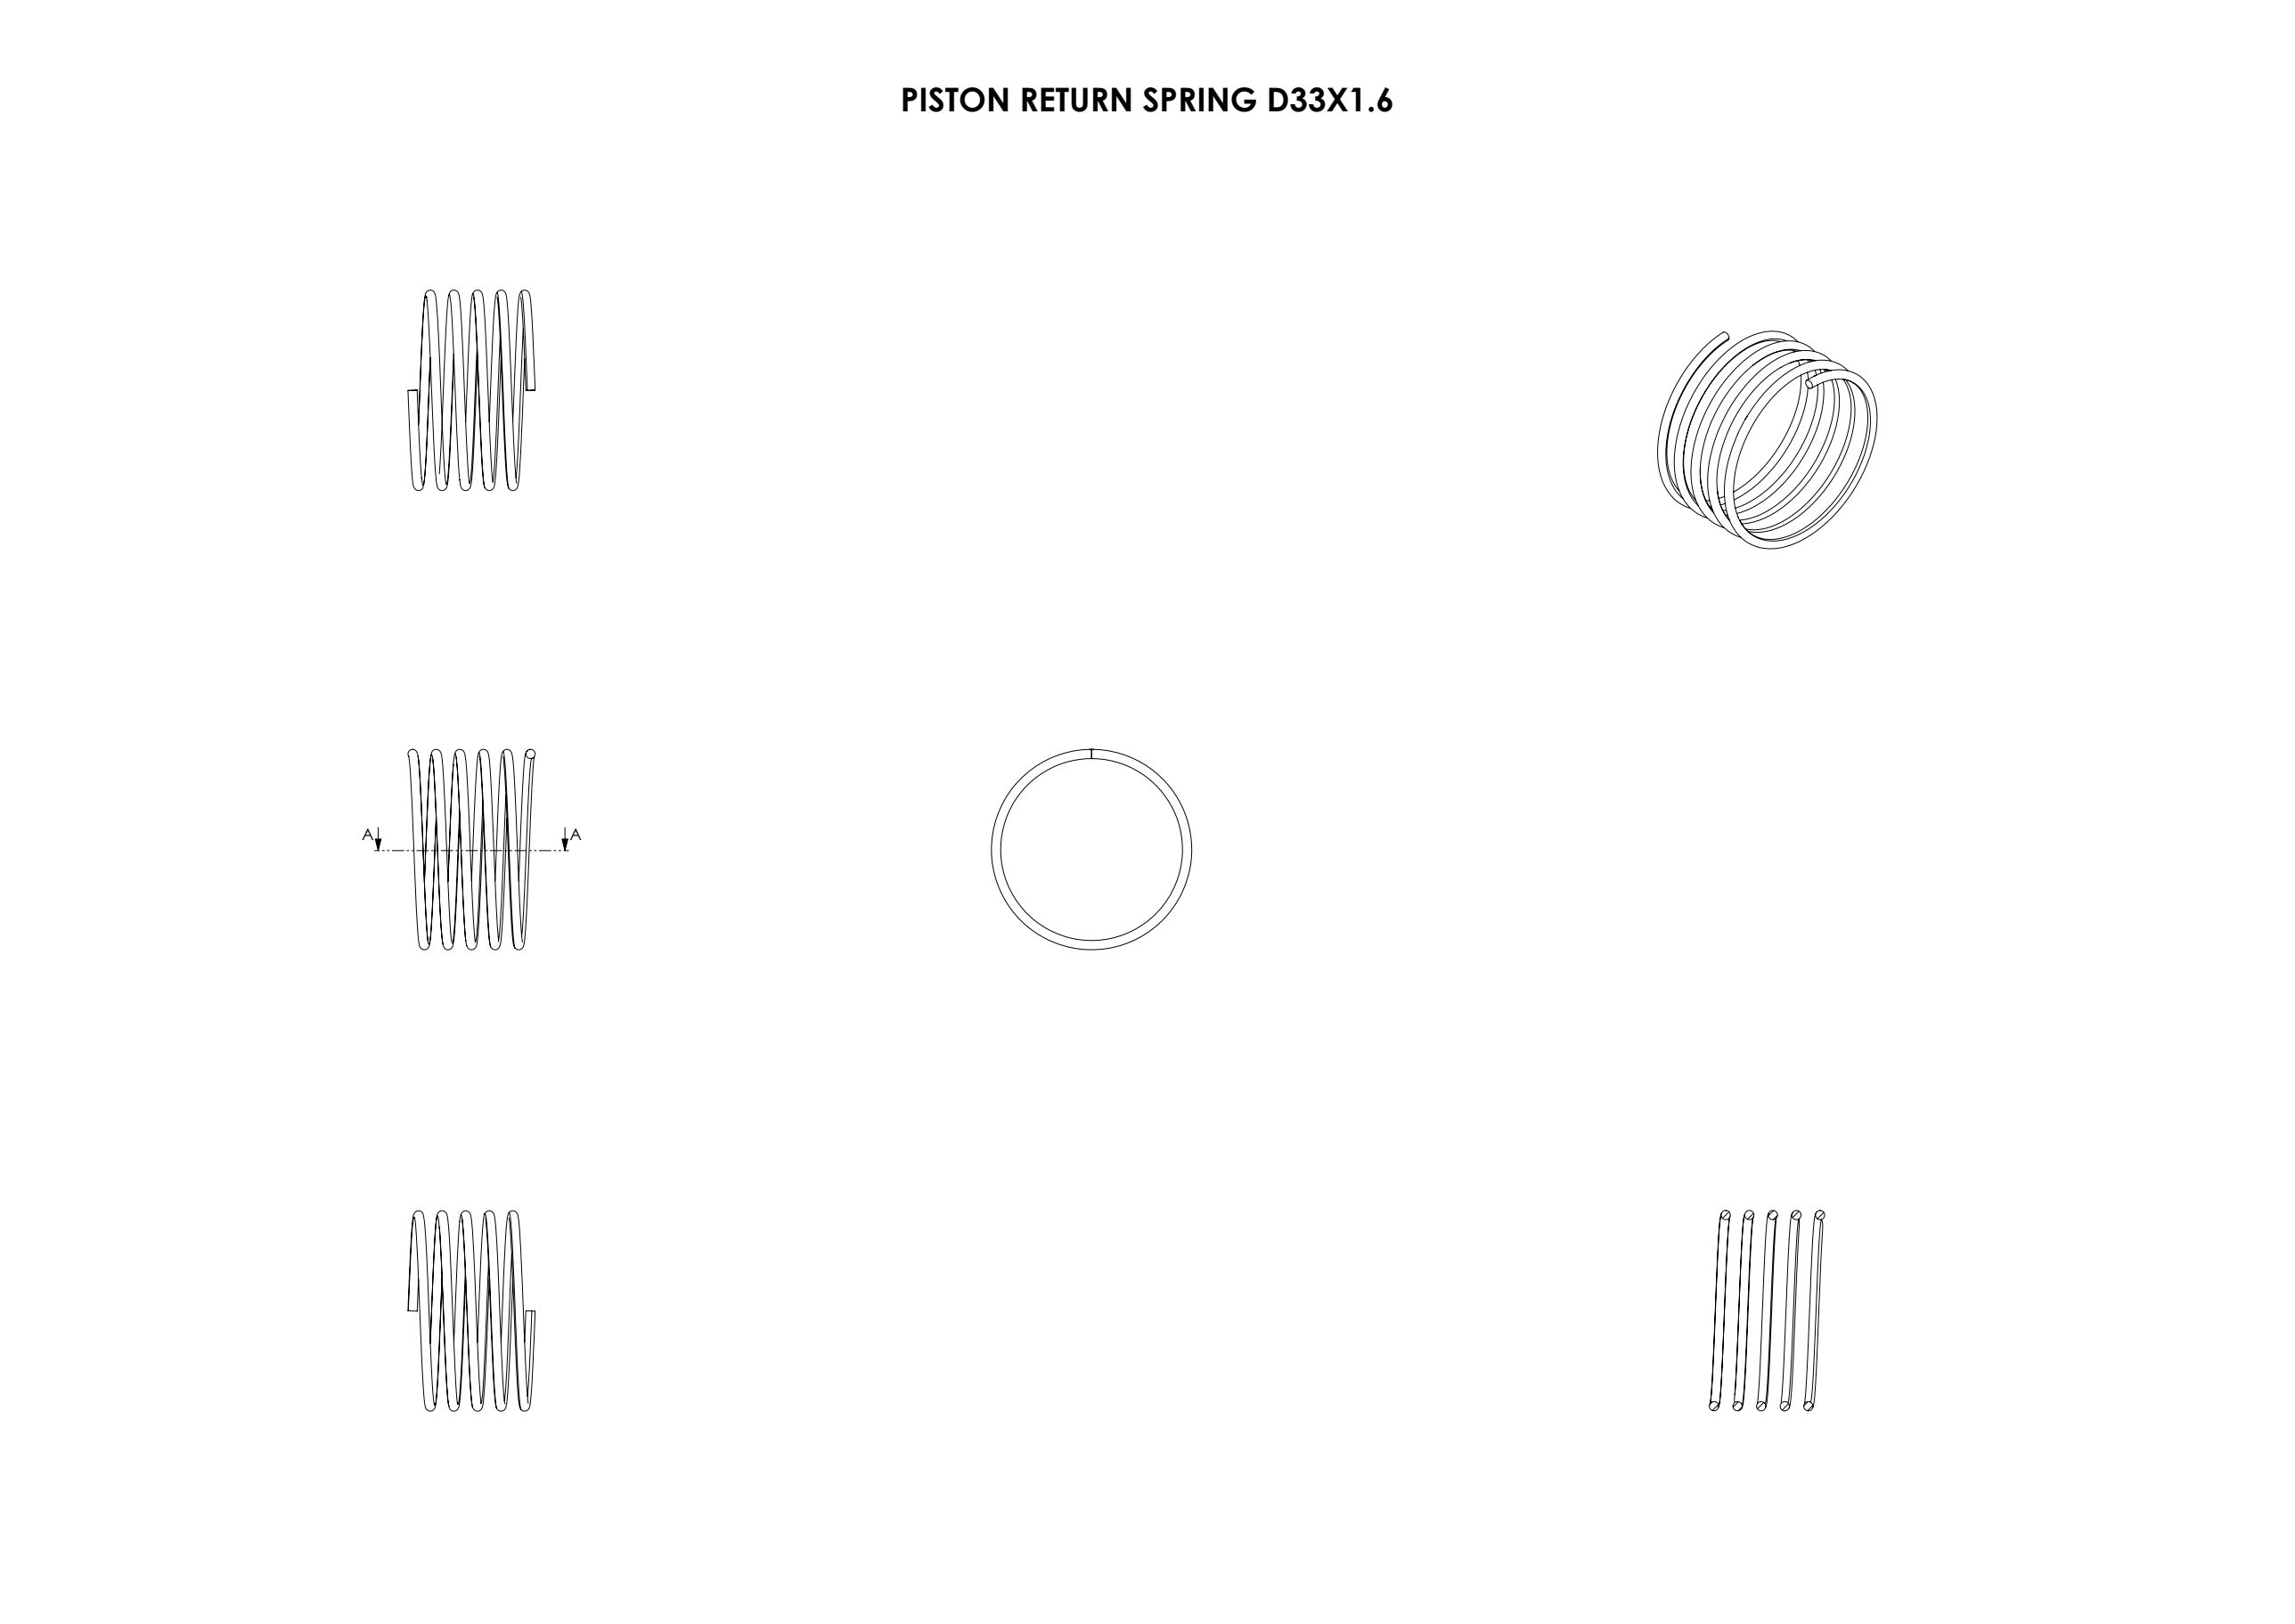
ISO-10303-21;
HEADER;
/* Generated by software containing ST-Developer
 * from STEP Tools, Inc. (www.steptools.com) 
 */

FILE_DESCRIPTION(
/* description */ (''),
/* implementation_level */ '2;1');

FILE_NAME(
/* name */ '04_Piston_Return_Spring_D33x1.6.step',
/* time_stamp */ '2026-10-26T03:55:20-07:00',
/* author */ (''),
/* organization */ (''),
/* preprocessor_version */ 'ST-DEVELOPER v20.2',
/* originating_system */ 'Autodesk Translation Framework v15.15.0.0',
/* authorisation */ '');

FILE_SCHEMA (('AUTOMOTIVE_DESIGN { 1 0 10303 214 3 1 1 }'));
ENDSEC;

DATA;
#10=MECHANICAL_DESIGN_GEOMETRIC_PRESENTATION_REPRESENTATION('',(#178),#45236);
#138=SHAPE_REPRESENTATION_RELATIONSHIP('SRR','None',#45317,#158);
#158=ADVANCED_BREP_SHAPE_REPRESENTATION('',(#198),#45219);
#178=STYLED_ITEM('',(#45484),#198);
#198=MANIFOLD_SOLID_BREP('Body1',#16520);
#484=B_SPLINE_CURVE_WITH_KNOTS('',3,(#32149,#32150,#32151,#32152,#32153,
#32154,#32155,#32156,#32157,#32158,#32159,#32160,#32161,#32162,#32163,#32164,
#32165,#32166,#32167,#32168,#32169,#32170,#32171,#32172,#32173,#32174,#32175,
#32176,#32177,#32178,#32179,#32180,#32181,#32182,#32183,#32184,#32185,#32186,
#32187,#32188,#32189,#32190,#32191,#32192,#32193,#32194,#32195,#32196,#32197,
#32198,#32199,#32200,#32201,#32202,#32203,#32204,#32205,#32206,#32207,#32208,
#32209,#32210,#32211,#32212,#32213,#32214,#32215,#32216,#32217,#32218,#32219,
#32220,#32221,#32222,#32223),.UNSPECIFIED.,.F.,.F.,(4,1,1,1,1,1,1,1,1,1,
1,1,1,1,1,1,1,1,1,1,1,1,1,1,1,1,1,1,1,1,1,1,1,1,1,1,1,1,1,1,1,1,1,1,1,1,
1,1,1,1,1,1,1,1,1,1,1,1,1,1,1,1,1,1,1,1,1,1,1,1,1,1,4),(0.,0.00892857142857143,
0.0178571428571429,0.0357142857142857,0.0535714285714286,0.0714285714285714,
0.0892857142857143,0.107142857142857,0.116071428571429,0.125,0.133928571428571,
0.142857142857143,0.154761904761905,0.166666666666667,0.178571428571429,
0.19047619047619,0.202380952380952,0.214285714285714,0.232142857142857,
0.25,0.267857142857143,0.285714285714286,0.303571428571429,0.321428571428571,
0.339285714285714,0.357142857142857,0.376984126984127,0.380952380952381,
0.392857142857143,0.404761904761905,0.416666666666667,0.428571428571429,
0.44047619047619,0.452380952380952,0.464285714285714,0.476190476190476,
0.492063492063492,0.5,0.517857142857143,0.535714285714286,0.553571428571429,
0.571428571428571,0.589285714285714,0.607142857142857,0.625,0.642857142857143,
0.654761904761905,0.666666666666667,0.678571428571428,0.69047619047619,
0.702380952380952,0.714285714285714,0.726190476190476,0.738095238095238,
0.75,0.761904761904762,0.773809523809524,0.785714285714286,0.797619047619047,
0.809523809523809,0.821428571428571,0.833333333333333,0.845238095238095,
0.857142857142857,0.875,0.892857142857143,0.910714285714286,0.928571428571429,
0.946428571428571,0.964285714285714,0.982142857142857,0.991071428571429,
1.),.UNSPECIFIED.);
#857=B_SPLINE_SURFACE_WITH_KNOTS('',3,3,((#31396,#31397,#31398,#31399,#31400,
#31401,#31402,#31403,#31404,#31405,#31406,#31407,#31408,#31409,#31410,#31411,
#31412,#31413,#31414,#31415,#31416,#31417,#31418,#31419,#31420,#31421,#31422,
#31423,#31424,#31425,#31426,#31427,#31428,#31429,#31430,#31431,#31432,#31433,
#31434,#31435,#31436,#31437,#31438,#31439,#31440,#31441,#31442,#31443,#31444,
#31445,#31446,#31447,#31448,#31449,#31450,#31451,#31452,#31453,#31454,#31455,
#31456,#31457,#31458,#31459,#31460,#31461,#31462,#31463,#31464,#31465,#31466,
#31467,#31468,#31469,#31470),(#31471,#31472,#31473,#31474,#31475,#31476,
#31477,#31478,#31479,#31480,#31481,#31482,#31483,#31484,#31485,#31486,#31487,
#31488,#31489,#31490,#31491,#31492,#31493,#31494,#31495,#31496,#31497,#31498,
#31499,#31500,#31501,#31502,#31503,#31504,#31505,#31506,#31507,#31508,#31509,
#31510,#31511,#31512,#31513,#31514,#31515,#31516,#31517,#31518,#31519,#31520,
#31521,#31522,#31523,#31524,#31525,#31526,#31527,#31528,#31529,#31530,#31531,
#31532,#31533,#31534,#31535,#31536,#31537,#31538,#31539,#31540,#31541,#31542,
#31543,#31544,#31545),(#31546,#31547,#31548,#31549,#31550,#31551,#31552,
#31553,#31554,#31555,#31556,#31557,#31558,#31559,#31560,#31561,#31562,#31563,
#31564,#31565,#31566,#31567,#31568,#31569,#31570,#31571,#31572,#31573,#31574,
#31575,#31576,#31577,#31578,#31579,#31580,#31581,#31582,#31583,#31584,#31585,
#31586,#31587,#31588,#31589,#31590,#31591,#31592,#31593,#31594,#31595,#31596,
#31597,#31598,#31599,#31600,#31601,#31602,#31603,#31604,#31605,#31606,#31607,
#31608,#31609,#31610,#31611,#31612,#31613,#31614,#31615,#31616,#31617,#31618,
#31619,#31620),(#31621,#31622,#31623,#31624,#31625,#31626,#31627,#31628,
#31629,#31630,#31631,#31632,#31633,#31634,#31635,#31636,#31637,#31638,#31639,
#31640,#31641,#31642,#31643,#31644,#31645,#31646,#31647,#31648,#31649,#31650,
#31651,#31652,#31653,#31654,#31655,#31656,#31657,#31658,#31659,#31660,#31661,
#31662,#31663,#31664,#31665,#31666,#31667,#31668,#31669,#31670,#31671,#31672,
#31673,#31674,#31675,#31676,#31677,#31678,#31679,#31680,#31681,#31682,#31683,
#31684,#31685,#31686,#31687,#31688,#31689,#31690,#31691,#31692,#31693,#31694,
#31695),(#31696,#31697,#31698,#31699,#31700,#31701,#31702,#31703,#31704,
#31705,#31706,#31707,#31708,#31709,#31710,#31711,#31712,#31713,#31714,#31715,
#31716,#31717,#31718,#31719,#31720,#31721,#31722,#31723,#31724,#31725,#31726,
#31727,#31728,#31729,#31730,#31731,#31732,#31733,#31734,#31735,#31736,#31737,
#31738,#31739,#31740,#31741,#31742,#31743,#31744,#31745,#31746,#31747,#31748,
#31749,#31750,#31751,#31752,#31753,#31754,#31755,#31756,#31757,#31758,#31759,
#31760,#31761,#31762,#31763,#31764,#31765,#31766,#31767,#31768,#31769,#31770),
(#31771,#31772,#31773,#31774,#31775,#31776,#31777,#31778,#31779,#31780,
#31781,#31782,#31783,#31784,#31785,#31786,#31787,#31788,#31789,#31790,#31791,
#31792,#31793,#31794,#31795,#31796,#31797,#31798,#31799,#31800,#31801,#31802,
#31803,#31804,#31805,#31806,#31807,#31808,#31809,#31810,#31811,#31812,#31813,
#31814,#31815,#31816,#31817,#31818,#31819,#31820,#31821,#31822,#31823,#31824,
#31825,#31826,#31827,#31828,#31829,#31830,#31831,#31832,#31833,#31834,#31835,
#31836,#31837,#31838,#31839,#31840,#31841,#31842,#31843,#31844,#31845),
(#31846,#31847,#31848,#31849,#31850,#31851,#31852,#31853,#31854,#31855,
#31856,#31857,#31858,#31859,#31860,#31861,#31862,#31863,#31864,#31865,#31866,
#31867,#31868,#31869,#31870,#31871,#31872,#31873,#31874,#31875,#31876,#31877,
#31878,#31879,#31880,#31881,#31882,#31883,#31884,#31885,#31886,#31887,#31888,
#31889,#31890,#31891,#31892,#31893,#31894,#31895,#31896,#31897,#31898,#31899,
#31900,#31901,#31902,#31903,#31904,#31905,#31906,#31907,#31908,#31909,#31910,
#31911,#31912,#31913,#31914,#31915,#31916,#31917,#31918,#31919,#31920),
(#31921,#31922,#31923,#31924,#31925,#31926,#31927,#31928,#31929,#31930,
#31931,#31932,#31933,#31934,#31935,#31936,#31937,#31938,#31939,#31940,#31941,
#31942,#31943,#31944,#31945,#31946,#31947,#31948,#31949,#31950,#31951,#31952,
#31953,#31954,#31955,#31956,#31957,#31958,#31959,#31960,#31961,#31962,#31963,
#31964,#31965,#31966,#31967,#31968,#31969,#31970,#31971,#31972,#31973,#31974,
#31975,#31976,#31977,#31978,#31979,#31980,#31981,#31982,#31983,#31984,#31985,
#31986,#31987,#31988,#31989,#31990,#31991,#31992,#31993,#31994,#31995),
(#31996,#31997,#31998,#31999,#32000,#32001,#32002,#32003,#32004,#32005,
#32006,#32007,#32008,#32009,#32010,#32011,#32012,#32013,#32014,#32015,#32016,
#32017,#32018,#32019,#32020,#32021,#32022,#32023,#32024,#32025,#32026,#32027,
#32028,#32029,#32030,#32031,#32032,#32033,#32034,#32035,#32036,#32037,#32038,
#32039,#32040,#32041,#32042,#32043,#32044,#32045,#32046,#32047,#32048,#32049,
#32050,#32051,#32052,#32053,#32054,#32055,#32056,#32057,#32058,#32059,#32060,
#32061,#32062,#32063,#32064,#32065,#32066,#32067,#32068,#32069,#32070),
(#32071,#32072,#32073,#32074,#32075,#32076,#32077,#32078,#32079,#32080,
#32081,#32082,#32083,#32084,#32085,#32086,#32087,#32088,#32089,#32090,#32091,
#32092,#32093,#32094,#32095,#32096,#32097,#32098,#32099,#32100,#32101,#32102,
#32103,#32104,#32105,#32106,#32107,#32108,#32109,#32110,#32111,#32112,#32113,
#32114,#32115,#32116,#32117,#32118,#32119,#32120,#32121,#32122,#32123,#32124,
#32125,#32126,#32127,#32128,#32129,#32130,#32131,#32132,#32133,#32134,#32135,
#32136,#32137,#32138,#32139,#32140,#32141,#32142,#32143,#32144,#32145)),
 .UNSPECIFIED.,.T.,.F.,.F.,(4,1,1,1,1,1,1,4),(4,1,1,1,1,1,1,1,1,1,1,1,1,
1,1,1,1,1,1,1,1,1,1,1,1,1,1,1,1,1,1,1,1,1,1,1,1,1,1,1,1,1,1,1,1,1,1,1,1,
1,1,1,1,1,1,1,1,1,1,1,1,1,1,1,1,1,1,1,1,1,1,1,4),(-3.14159265358979,-2.24399475256414,
-1.34639685153848,-0.448798950512828,0.448798950512828,1.34639685153848,
2.24399475256414,3.14159265358979),(0.,0.00892857142857143,0.0178571428571429,
0.0357142857142857,0.0535714285714286,0.0714285714285714,0.0892857142857143,
0.107142857142857,0.116071428571429,0.125,0.133928571428571,0.142857142857143,
0.154761904761905,0.166666666666667,0.178571428571429,0.19047619047619,
0.202380952380952,0.214285714285714,0.232142857142857,0.25,0.267857142857143,
0.285714285714286,0.303571428571429,0.321428571428571,0.339285714285714,
0.357142857142857,0.376984126984127,0.380952380952381,0.392857142857143,
0.404761904761905,0.416666666666667,0.428571428571429,0.44047619047619,
0.452380952380952,0.464285714285714,0.476190476190476,0.492063492063492,
0.5,0.517857142857143,0.535714285714286,0.553571428571429,0.571428571428571,
0.589285714285714,0.607142857142857,0.625,0.642857142857143,0.654761904761905,
0.666666666666667,0.678571428571428,0.69047619047619,0.702380952380952,
0.714285714285714,0.726190476190476,0.738095238095238,0.75,0.761904761904762,
0.773809523809524,0.785714285714286,0.797619047619047,0.809523809523809,
0.821428571428571,0.833333333333333,0.845238095238095,0.857142857142857,
0.875,0.892857142857143,0.910714285714286,0.928571428571429,0.946428571428571,
0.964285714285714,0.982142857142857,0.991071428571429,1.),.UNSPECIFIED.);
#1130=PLANE('',#17150);
#1131=PLANE('',#17151);
#2088=FACE_OUTER_BOUND('',#3086,.T.);
#2089=FACE_OUTER_BOUND('',#3087,.T.);
#2090=FACE_OUTER_BOUND('',#3088,.T.);
#3086=EDGE_LOOP('',(#12128,#12129,#12130,#12131));
#3087=EDGE_LOOP('',(#12132));
#3088=EDGE_LOOP('',(#12133));
#6661=CIRCLE('',#17148,0.8);
#6662=CIRCLE('',#17149,0.8);
#7377=VERTEX_POINT('',#32146);
#7378=VERTEX_POINT('',#32148);
#9127=EDGE_CURVE('',#7377,#7377,#6661,.T.);
#9128=EDGE_CURVE('',#7377,#7378,#484,.T.);
#9129=EDGE_CURVE('',#7378,#7378,#6662,.T.);
#12128=ORIENTED_EDGE('',*,*,#9127,.T.);
#12129=ORIENTED_EDGE('',*,*,#9128,.T.);
#12130=ORIENTED_EDGE('',*,*,#9129,.F.);
#12131=ORIENTED_EDGE('',*,*,#9128,.F.);
#12132=ORIENTED_EDGE('',*,*,#9129,.T.);
#12133=ORIENTED_EDGE('',*,*,#9127,.F.);
#15816=ADVANCED_FACE('',(#2088),#857,.T.);
#15817=ADVANCED_FACE('',(#2089),#1130,.T.);
#15818=ADVANCED_FACE('',(#2090),#1131,.F.);
#16520=CLOSED_SHELL('',(#15816,#15817,#15818));
#17147=AXIS2_PLACEMENT_3D('',#31395,#19181,#19182);
#17148=AXIS2_PLACEMENT_3D('',#32147,#19183,#19184);
#17149=AXIS2_PLACEMENT_3D('',#32224,#19185,#19186);
#17150=AXIS2_PLACEMENT_3D('',#32225,#19187,#19188);
#17151=AXIS2_PLACEMENT_3D('',#32226,#19189,#19190);
#19181=DIRECTION('axis',(0.,0.,1.));
#19182=DIRECTION('refdir',(1.,0.,0.));
#19183=DIRECTION('center_axis',(0.0385833407296796,-0.00185275719821836,
0.99925366804876));
#19184=DIRECTION('ref_axis',(-0.998103575378143,0.0479285502208167,0.0386277994596909));
#19185=DIRECTION('center_axis',(0.0385833409756958,0.0018527571775933,0.999253668039299));
#19186=DIRECTION('ref_axis',(-0.285673463027164,0.95828233937443,0.00925367846524069));
#19187=DIRECTION('center_axis',(0.0385833409756958,0.0018527571775933,0.999253668039299));
#19188=DIRECTION('ref_axis',(-0.285673463027164,0.95828233937443,0.00925367846524068));
#19189=DIRECTION('center_axis',(0.0385833407296796,-0.00185275719821836,
0.99925366804876));
#19190=DIRECTION('ref_axis',(-0.998103575378143,0.0479285502208167,0.0386277994596909));
#31395=CARTESIAN_POINT('',(0.,0.,0.));
#31396=CARTESIAN_POINT('Ctrl Pts',(69.6184828603025,16.4616571598233,-0.030902239567753));
#31397=CARTESIAN_POINT('Ctrl Pts',(69.6789219655699,16.458754897209,1.53438465601481));
#31398=CARTESIAN_POINT('Ctrl Pts',(69.7997830801149,16.0266321943109,4.57501994136558));
#31399=CARTESIAN_POINT('Ctrl Pts',(70.0414349064678,13.4941722421641,10.2617903021912));
#31400=CARTESIAN_POINT('Ctrl Pts',(70.3432064666604,7.54051932200945,15.5847054098009));
#31401=CARTESIAN_POINT('Ctrl Pts',(70.7049768750637,-1.90873983484295,17.1894487135762));
#31402=CARTESIAN_POINT('Ctrl Pts',(71.0663492060979,-10.7475553396686,13.525924310196));
#31403=CARTESIAN_POINT('Ctrl Pts',(71.4273437518671,-16.2818464768058,5.72657424978343));
#31404=CARTESIAN_POINT('Ctrl Pts',(71.7278512234343,-16.7210289894503,-2.21659997283488));
#31405=CARTESIAN_POINT('Ctrl Pts',(71.9680675578449,-14.5106197428725,-7.98557322489482));
#31406=CARTESIAN_POINT('Ctrl Pts',(72.1481344157904,-11.7288725172833,-11.6852538002611));
#31407=CARTESIAN_POINT('Ctrl Pts',(72.328106524648,-8.03024824250695,-14.4669696417765));
#31408=CARTESIAN_POINT('Ctrl Pts',(72.5279702250768,-3.22977654241172,-16.300670274406));
#31409=CARTESIAN_POINT('Ctrl Pts',(72.7476856540044,2.4587525001183,-16.5141747132305));
#31410=CARTESIAN_POINT('Ctrl Pts',(72.9872078330289,8.31673840998305,-14.4634243432854));
#31411=CARTESIAN_POINT('Ctrl Pts',(73.2265632969346,13.0163496494046,-10.4182667032949));
#31412=CARTESIAN_POINT('Ctrl Pts',(73.4657526686465,15.9141590581627,-4.93897396144999));
#31413=CARTESIAN_POINT('Ctrl Pts',(73.7047766516472,16.6034312776959,1.21397241511146));
#31414=CARTESIAN_POINT('Ctrl Pts',(73.9834458021771,14.7409225736484,8.19195097348461));
#31415=CARTESIAN_POINT('Ctrl Pts',(74.301651818573,9.13086318160831,14.4766680019069));
#31416=CARTESIAN_POINT('Ctrl Pts',(74.6592672763964,0.0266353994119735,
17.0966775050227));
#31417=CARTESIAN_POINT('Ctrl Pts',(75.016519558125,-9.06348425632334,14.4765973593132));
#31418=CARTESIAN_POINT('Ctrl Pts',(75.3734117874807,-15.3610417662207,7.42742367726323));
#31419=CARTESIAN_POINT('Ctrl Pts',(75.7299471567895,-16.9418739975217,-1.88122771580553));
#31420=CARTESIAN_POINT('Ctrl Pts',(76.0861289312927,-13.3290621410899,-10.5975142741848));
#31421=CARTESIAN_POINT('Ctrl Pts',(76.4419606933661,-5.64617345782912,-16.0463992053949));
#31422=CARTESIAN_POINT('Ctrl Pts',(76.810612386967,4.11087115606672,-16.6005218369866));
#31423=CARTESIAN_POINT('Ctrl Pts',(77.0868204963524,10.4484384772329,-12.8295775485076));
#31424=CARTESIAN_POINT('Ctrl Pts',(77.3234199677928,14.1464940116618,-8.0565595801055));
#31425=CARTESIAN_POINT('Ctrl Pts',(77.5073642434964,16.0558684975652,-3.69288655028273));
#31426=CARTESIAN_POINT('Ctrl Pts',(77.743715642047,16.2835727900373,2.42892269363191));
#31427=CARTESIAN_POINT('Ctrl Pts',(77.9799198273595,14.2624210045081,8.20410639070391));
#31428=CARTESIAN_POINT('Ctrl Pts',(78.2159782861261,10.2721221270508,12.8404255794219));
#31429=CARTESIAN_POINT('Ctrl Pts',(78.451892297019,4.86870939460828,15.6955819848942));
#31430=CARTESIAN_POINT('Ctrl Pts',(78.687663274949,-1.20342672163651,16.3804065631851));
#31431=CARTESIAN_POINT('Ctrl Pts',(78.923292730736,-7.09646797598974,14.7976258939457));
#31432=CARTESIAN_POINT('Ctrl Pts',(79.1849474554113,-12.559397153018,10.7746599228106));
#31433=CARTESIAN_POINT('Ctrl Pts',(79.4202749429787,-15.5097121162534,5.34934186422077));
#31434=CARTESIAN_POINT('Ctrl Pts',(79.6946643695902,-16.3852200323318,-1.64037324259347));
#31435=CARTESIAN_POINT('Ctrl Pts',(79.9819403068823,-14.2884064522935,-8.94742064680176));
#31436=CARTESIAN_POINT('Ctrl Pts',(80.3342067288376,-7.3260467326971,-15.165426706738));
#31437=CARTESIAN_POINT('Ctrl Pts',(80.6861788812633,1.86167912032264,-16.7248261450382));
#31438=CARTESIAN_POINT('Ctrl Pts',(81.037862268153,10.4673895230379,-13.1602039003653));
#31439=CARTESIAN_POINT('Ctrl Pts',(81.3892625213115,15.8514527926196,-5.5687461546451));
#31440=CARTESIAN_POINT('Ctrl Pts',(81.7403859218982,16.3720606810702,3.71439472873355));
#31441=CARTESIAN_POINT('Ctrl Pts',(82.0912385240458,11.8761863054331,11.8495550298708));
#31442=CARTESIAN_POINT('Ctrl Pts',(82.4028723251709,4.65229996881944,15.8345467687591));
#31443=CARTESIAN_POINT('Ctrl Pts',(82.6753839687717,-2.4057965557233,16.0912478601411));
#31444=CARTESIAN_POINT('Ctrl Pts',(82.9088524431066,-8.11448174868296,14.0955831155642));
#31445=CARTESIAN_POINT('Ctrl Pts',(83.1422098352473,-12.6971950976412,10.1502287241044));
#31446=CARTESIAN_POINT('Ctrl Pts',(83.3754581634701,-15.522088392645,4.8081952387983));
#31447=CARTESIAN_POINT('Ctrl Pts',(83.6085992893649,-16.1966474690964,-1.19488542166675));
#31448=CARTESIAN_POINT('Ctrl Pts',(83.8416352233784,-14.6339538883274,-7.02670369688337));
#31449=CARTESIAN_POINT('Ctrl Pts',(84.0745679545012,-11.0497598473816,-11.8824317127295));
#31450=CARTESIAN_POINT('Ctrl Pts',(84.3073996737489,-5.94248428783527,-15.09263970399));
#31451=CARTESIAN_POINT('Ctrl Pts',(84.540132268385,-0.0171665032603614,
-16.2129461632812));
#31452=CARTESIAN_POINT('Ctrl Pts',(84.7727680106188,5.90520262635639,-15.0923025294507));
#31453=CARTESIAN_POINT('Ctrl Pts',(85.0053088744204,11.0065171159269,-11.8864785100097));
#31454=CARTESIAN_POINT('Ctrl Pts',(85.2377570340819,14.5833427924651,-7.04062680693156));
#31455=CARTESIAN_POINT('Ctrl Pts',(85.4701144791861,16.1401640578478,-1.22533588346504));
#31456=CARTESIAN_POINT('Ctrl Pts',(85.7023835299595,15.4662929248669,4.7550040735545));
#31457=CARTESIAN_POINT('Ctrl Pts',(85.9345662446591,12.6553888178413,10.0730373304554));
#31458=CARTESIAN_POINT('Ctrl Pts',(86.1666649327954,8.09679983295076,13.9966583914468));
#31459=CARTESIAN_POINT('Ctrl Pts',(86.3986815381799,2.42358552200963,15.9794357678464));
#31460=CARTESIAN_POINT('Ctrl Pts',(86.6692750541127,-4.58486198073758,15.7239726419428));
#31461=CARTESIAN_POINT('Ctrl Pts',(86.9783943834765,-11.7499252678846,11.7698005968098));
#31462=CARTESIAN_POINT('Ctrl Pts',(87.3259902517892,-16.2024151439095,3.70954956442589));
#31463=CARTESIAN_POINT('Ctrl Pts',(87.6734207471648,-15.6862303609498,-5.47622167055361));
#31464=CARTESIAN_POINT('Ctrl Pts',(88.0207132272952,-10.3628479251535,-12.9771513909202));
#31465=CARTESIAN_POINT('Ctrl Pts',(88.3678323138933,-1.8703041859877,-16.4954810466909));
#31466=CARTESIAN_POINT('Ctrl Pts',(88.7148821316246,7.193051660985,-14.9532751855446));
#31467=CARTESIAN_POINT('Ctrl Pts',(89.003856786706,12.8943942592402,-9.85553205895293));
#31468=CARTESIAN_POINT('Ctrl Pts',(89.2351907747089,15.3179503044652,-4.41141050395984));
#31469=CARTESIAN_POINT('Ctrl Pts',(89.3506074633962,15.7305922894428,-1.50774141983879));
#31470=CARTESIAN_POINT('Ctrl Pts',(89.4085387704217,15.7333741285005,-0.00740294277221285));
#31471=CARTESIAN_POINT('Ctrl Pts',(69.6299635796842,16.7007411089511,-0.030902239567753));
#31472=CARTESIAN_POINT('Ctrl Pts',(69.6912334101605,16.6977989552313,1.55589925782231));
#31473=CARTESIAN_POINT('Ctrl Pts',(69.8138990070948,16.2591916609345,4.64186903714546));
#31474=CARTESIAN_POINT('Ctrl Pts',(70.0590053500828,13.6903812708504,10.4098634757414));
#31475=CARTESIAN_POINT('Ctrl Pts',(70.3651870367565,7.65014590609584,15.8105713921737));
#31476=CARTESIAN_POINT('Ctrl Pts',(70.7321817761829,-1.93568018811406,17.4381266158968));
#31477=CARTESIAN_POINT('Ctrl Pts',(71.098790206296,-10.902202057407,13.7218082112497));
#31478=CARTESIAN_POINT('Ctrl Pts',(71.4649915562623,-16.5161793686399,5.80994623870215));
#31479=CARTESIAN_POINT('Ctrl Pts',(71.7698338155353,-16.9616095340376,-2.24746365248745));
#31480=CARTESIAN_POINT('Ctrl Pts',(72.0134956355215,-14.7194966934706,-8.09911469764596));
#31481=CARTESIAN_POINT('Ctrl Pts',(72.1961430998093,-11.8979192255808,-11.8517332522967));
#31482=CARTESIAN_POINT('Ctrl Pts',(72.3786898054422,-8.14642913059767,-14.6731732353235));
#31483=CARTESIAN_POINT('Ctrl Pts',(72.5814069366342,-3.2774945734574,-16.5329935539285));
#31484=CARTESIAN_POINT('Ctrl Pts',(72.8042563013791,2.492037402214,-16.7494956008958));
#31485=CARTESIAN_POINT('Ctrl Pts',(73.0471841649293,8.43315113900825,-14.6695887137585));
#31486=CARTESIAN_POINT('Ctrl Pts',(73.2899316670396,13.1992567794014,-10.5671940850375));
#31487=CARTESIAN_POINT('Ctrl Pts',(73.5324951429592,16.1378423633534,-5.01067722190336));
#31488=CARTESIAN_POINT('Ctrl Pts',(73.7748792762995,16.8367888818105,1.22864251856273));
#31489=CARTESIAN_POINT('Ctrl Pts',(74.0574511370909,14.9481657499348,8.30419026726172));
#31490=CARTESIAN_POINT('Ctrl Pts',(74.3801042223558,9.25988647762291,14.6764058998477));
#31491=CARTESIAN_POINT('Ctrl Pts',(74.7426760471007,0.0297310386788871,
17.3325017860091));
#31492=CARTESIAN_POINT('Ctrl Pts',(75.104846156915,-9.18512009888459,14.6763349999953));
#31493=CARTESIAN_POINT('Ctrl Pts',(75.4666115601473,-15.5683097019005,7.53105835502853));
#31494=CARTESIAN_POINT('Ctrl Pts',(75.8279755375281,-17.1703047170958,-1.90331404102187));
#31495=CARTESIAN_POINT('Ctrl Pts',(76.188938501318,-13.5089512690439,-10.7361694860703));
#31496=CARTESIAN_POINT('Ctrl Pts',(76.5495030570368,-5.72407492543645,-16.2571081843157));
#31497=CARTESIAN_POINT('Ctrl Pts',(76.9230101424883,4.16106946480652,-16.8182717566536));
#31498=CARTESIAN_POINT('Ctrl Pts',(77.202818264229,10.5808314274358,-12.9982088799238));
#31499=CARTESIAN_POINT('Ctrl Pts',(77.4424552125793,14.3263048597699,-8.16392560339528));
#31500=CARTESIAN_POINT('Ctrl Pts',(77.6287702720463,16.2601131044503,-3.74422807442518));
#31501=CARTESIAN_POINT('Ctrl Pts',(77.8681200492692,16.4905653153525,2.45516469208262));
#31502=CARTESIAN_POINT('Ctrl Pts',(78.1073167318528,14.4438592167683,8.30318709138602));
#31503=CARTESIAN_POINT('Ctrl Pts',(78.3463319999749,10.4036277093244,12.9973204036373));
#31504=CARTESIAN_POINT('Ctrl Pts',(78.5851753685171,4.93332187654749,15.8877883112078));
#31505=CARTESIAN_POINT('Ctrl Pts',(78.8238536783697,-1.2133830481093,16.5809207741654));
#31506=CARTESIAN_POINT('Ctrl Pts',(79.0623433276802,-7.17782048654887,14.9789375723993));
#31507=CARTESIAN_POINT('Ctrl Pts',(79.3271592739995,-12.7064511092803,10.9074960661302));
#31508=CARTESIAN_POINT('Ctrl Pts',(79.5652827398898,-15.6916289014183,5.4178031995205));
#31509=CARTESIAN_POINT('Ctrl Pts',(79.842897654509,-16.577371391909,-1.65388631398067));
#31510=CARTESIAN_POINT('Ctrl Pts',(80.1335376112271,-14.4559690043196,-9.04592183069228));
#31511=CARTESIAN_POINT('Ctrl Pts',(80.4898408484177,-7.41398466215342,-15.3346562519615));
#31512=CARTESIAN_POINT('Ctrl Pts',(80.8457786444577,1.87672500454577,-16.9113054373767));
#31513=CARTESIAN_POINT('Ctrl Pts',(81.2013471369382,10.5769015012641,-13.3072352789264));
#31514=CARTESIAN_POINT('Ctrl Pts',(81.5565536242783,16.0187171293741,-5.63382944603668));
#31515=CARTESIAN_POINT('Ctrl Pts',(81.9114041755206,16.5444635000022,3.74727126004245));
#31516=CARTESIAN_POINT('Ctrl Pts',(82.2658984013975,12.0018869829841,11.9662350574611));
#31517=CARTESIAN_POINT('Ctrl Pts',(82.580705722997,4.7048385127119,15.9911824539821));
#31518=CARTESIAN_POINT('Ctrl Pts',(82.8559194126613,-2.42294966179176,16.2502803669511));
#31519=CARTESIAN_POINT('Ctrl Pts',(83.0916726679261,-8.18711284436968,14.2350674883706));
#31520=CARTESIAN_POINT('Ctrl Pts',(83.3272719462452,-12.8135954548322,10.2519305382705));
#31521=CARTESIAN_POINT('Ctrl Pts',(83.5627180336617,-15.6648270622522,4.85970543368255));
#31522=CARTESIAN_POINT('Ctrl Pts',(83.7980160722245,-16.3455482298039,-1.19867931322076));
#31523=CARTESIAN_POINT('Ctrl Pts',(84.0331762295264,-14.7685260231452,-7.08329288367993));
#31524=CARTESIAN_POINT('Ctrl Pts',(84.268196402248,-11.152406439379,-11.9821788257332));
#31525=CARTESIAN_POINT('Ctrl Pts',(84.5030544855061,-6.00074180238162,-15.220102481595));
#31526=CARTESIAN_POINT('Ctrl Pts',(84.7377942906585,-0.0247637862782051,
-16.349923638104));
#31527=CARTESIAN_POINT('Ctrl Pts',(84.9723852268477,5.94701813960035,-15.2197727933618));
#31528=CARTESIAN_POINT('Ctrl Pts',(85.2068382906793,11.0899618363975,-11.9877327276318));
#31529=CARTESIAN_POINT('Ctrl Pts',(85.4411634196362,14.69529952864,-7.10303215385319));
#31530=CARTESIAN_POINT('Ctrl Pts',(85.6753317373745,16.2641505061611,-1.24258983811037));
#31531=CARTESIAN_POINT('Ctrl Pts',(85.9093834453529,15.585023498085,4.78327339443017));
#31532=CARTESIAN_POINT('Ctrl Pts',(86.1433022075475,12.753189678752,10.1407102289761));
#31533=CARTESIAN_POINT('Ctrl Pts',(86.3770904163802,8.16161557939224,14.092613988289));
#31534=CARTESIAN_POINT('Ctrl Pts',(86.6107514938686,2.44850143153797,16.0892442032996));
#31535=CARTESIAN_POINT('Ctrl Pts',(86.8832033492737,-4.60774973811352,15.8319258548194));
#31536=CARTESIAN_POINT('Ctrl Pts',(87.1943932596932,-11.8200353832729,11.8513593361907));
#31537=CARTESIAN_POINT('Ctrl Pts',(87.5441993244538,-16.3001894463018,3.74019158563494));
#31538=CARTESIAN_POINT('Ctrl Pts',(87.8937391620268,-15.7805135997167,-5.50056638327167));
#31539=CARTESIAN_POINT('Ctrl Pts',(88.2430281368494,-10.4265102210085,-13.0439396213998));
#31540=CARTESIAN_POINT('Ctrl Pts',(88.5920456840267,-1.88797983749057,-16.5806798110945));
#31541=CARTESIAN_POINT('Ctrl Pts',(88.9408683355879,7.22126413171238,-15.0304223652045));
#31542=CARTESIAN_POINT('Ctrl Pts',(89.2312672507147,12.9500498613897,-9.90768422321171));
#31543=CARTESIAN_POINT('Ctrl Pts',(89.4636241947003,15.3843347561836,-4.4396343063962));
#31544=CARTESIAN_POINT('Ctrl Pts',(89.579568951633,15.7989939693362,-1.52285979480461));
#31545=CARTESIAN_POINT('Ctrl Pts',(89.6377374019334,15.8017871959225,-0.016379644123816));
#31546=CARTESIAN_POINT('Ctrl Pts',(69.4240531709196,17.1884297818141,-0.0220473507209931));
#31547=CARTESIAN_POINT('Ctrl Pts',(69.4870264995728,17.1854058267664,1.60887232745941));
#31548=CARTESIAN_POINT('Ctrl Pts',(69.6133825166773,16.7336094867537,4.78766921575342));
#31549=CARTESIAN_POINT('Ctrl Pts',(69.8655902618346,14.0901641326339,10.722743766396));
#31550=CARTESIAN_POINT('Ctrl Pts',(70.1808991871154,7.87082916461279,16.2850634142074));
#31551=CARTESIAN_POINT('Ctrl Pts',(70.5588258651904,-2.00097801197751,17.9608997165613));
#31552=CARTESIAN_POINT('Ctrl Pts',(70.9364976647261,-11.2379749124772,14.1333434106797));
#31553=CARTESIAN_POINT('Ctrl Pts',(71.3138189090291,-17.022765187301,5.98116984148052));
#31554=CARTESIAN_POINT('Ctrl Pts',(71.6279973568013,-17.4821577443558,-2.32283482661027));
#31555=CARTESIAN_POINT('Ctrl Pts',(71.8791587044794,-15.1710757913127,-8.35466252474748));
#31556=CARTESIAN_POINT('Ctrl Pts',(72.0674480802091,-12.2623824355508,-12.2232151758295));
#31557=CARTESIAN_POINT('Ctrl Pts',(72.2556517362955,-8.39465033453757,-15.1321399832916));
#31558=CARTESIAN_POINT('Ctrl Pts',(72.4646714233985,-3.37434570819596,-17.0498317563071));
#31559=CARTESIAN_POINT('Ctrl Pts',(72.6944730924827,2.57520497582538,-17.2731773805752));
#31560=CARTESIAN_POINT('Ctrl Pts',(72.9450091193642,8.70245453300236,-15.1282047436106));
#31561=CARTESIAN_POINT('Ctrl Pts',(73.1953872307492,13.6184515692381,-10.8968875890289));
#31562=CARTESIAN_POINT('Ctrl Pts',(73.4456025501822,16.6498267526876,-5.16509270015882));
#31563=CARTESIAN_POINT('Ctrl Pts',(73.6956575744498,17.3709549472363,1.27172072423803));
#31564=CARTESIAN_POINT('Ctrl Pts',(73.9871985164346,15.4224581181395,8.57192585469278));
#31565=CARTESIAN_POINT('Ctrl Pts',(74.3201228056949,9.55312842944366,15.147214623983));
#31566=CARTESIAN_POINT('Ctrl Pts',(74.694282229127,0.0278963775676262,17.8884110165378));
#31567=CARTESIAN_POINT('Ctrl Pts',(75.0680626554788,-9.48257511274735,15.1471822094838));
#31568=CARTESIAN_POINT('Ctrl Pts',(75.4414566077462,-16.0711692555847,7.77218199232533));
#31569=CARTESIAN_POINT('Ctrl Pts',(75.8144609438332,-17.7249238578617,-1.96628250261766));
#31570=CARTESIAN_POINT('Ctrl Pts',(76.1870708489347,-13.9454473073086,-11.0843892045722));
#31571=CARTESIAN_POINT('Ctrl Pts',(76.5592825554438,-5.90895378486479,-16.7838920968456));
#31572=CARTESIAN_POINT('Ctrl Pts',(76.944862466462,4.29597064015474,-17.3632704575972));
#31573=CARTESIAN_POINT('Ctrl Pts',(77.233714179634,10.9234377023668,-13.419633731763));
#31574=CARTESIAN_POINT('Ctrl Pts',(77.481110180057,14.7902150666366,-8.42881512726714));
#31575=CARTESIAN_POINT('Ctrl Pts',(77.6734420678579,16.786574081098,-3.86622860214854));
#31576=CARTESIAN_POINT('Ctrl Pts',(77.9205334101491,17.0245270944407,2.53374212629342));
#31577=CARTESIAN_POINT('Ctrl Pts',(78.1674468691423,14.9117140996151,8.57064368391211));
#31578=CARTESIAN_POINT('Ctrl Pts',(78.4141712309578,10.7410900027972,13.4163330220923));
#31579=CARTESIAN_POINT('Ctrl Pts',(78.6607089908048,5.09438525439352,16.3999664439789));
#31580=CARTESIAN_POINT('Ctrl Pts',(78.907060486491,-1.2501642558568,17.115417594678));
#31581=CARTESIAN_POINT('Ctrl Pts',(79.1532182906523,-7.40645575193075,15.4618484055836));
#31582=CARTESIAN_POINT('Ctrl Pts',(79.4265206417368,-13.1124389073509,11.2597518864601));
#31583=CARTESIAN_POINT('Ctrl Pts',(79.6722671305222,-16.1931862086824,5.59418186052905));
#31584=CARTESIAN_POINT('Ctrl Pts',(79.9587481865963,-17.107208902634,-1.70351483576795));
#31585=CARTESIAN_POINT('Ctrl Pts',(80.2586234108375,-14.9181543555872,-9.33083857880673));
#31586=CARTESIAN_POINT('Ctrl Pts',(80.6262139427276,-7.65267738846512,-15.8189271434239));
#31587=CARTESIAN_POINT('Ctrl Pts',(80.993369645609,1.93135544061078,-17.4451185003386));
#31588=CARTESIAN_POINT('Ctrl Pts',(81.3600870123395,10.9046720730943,-13.7276751808303));
#31589=CARTESIAN_POINT('Ctrl Pts',(81.7263654465945,16.516198667685,-5.81456179905747));
#31590=CARTESIAN_POINT('Ctrl Pts',(82.0922035782066,17.058047794173,3.85756185847759));
#31591=CARTESIAN_POINT('Ctrl Pts',(82.4575998851323,12.3753093119527,12.3295869826222));
#31592=CARTESIAN_POINT('Ctrl Pts',(82.7820047281608,4.85519133781646,16.4773647557847));
#31593=CARTESIAN_POINT('Ctrl Pts',(83.06556961557,-2.48914093741938,16.7442492288014));
#31594=CARTESIAN_POINT('Ctrl Pts',(83.3084289758973,-8.42735448041435,14.6681468183089));
#31595=CARTESIAN_POINT('Ctrl Pts',(83.5510909458127,-13.1926413221872,10.5653533262531));
#31596=CARTESIAN_POINT('Ctrl Pts',(83.7935551432849,-16.1289593487553,5.01216886238094));
#31597=CARTESIAN_POINT('Ctrl Pts',(84.0358223101127,-16.8297188132406,-1.22589245673049));
#31598=CARTESIAN_POINT('Ctrl Pts',(84.2778927289577,-15.2062416115988,-7.28372473114384));
#31599=CARTESIAN_POINT('Ctrl Pts',(84.519766488978,-11.484320451343,-12.3256879562995));
#31600=CARTESIAN_POINT('Ctrl Pts',(84.761441837939,-6.18293902347355,-15.6576372355493));
#31601=CARTESIAN_POINT('Ctrl Pts',(85.0029217884757,-0.0349046563979193,
-16.8198288925798));
#31602=CARTESIAN_POINT('Ctrl Pts',(85.2442044100241,6.10753989381876,-15.6573076159067));
#31603=CARTESIAN_POINT('Ctrl Pts',(85.4852907630462,11.3961830117023,-12.3334882012418));
#31604=CARTESIAN_POINT('Ctrl Pts',(85.726181088518,15.1027170540795,-7.31150778152954));
#31605=CARTESIAN_POINT('Ctrl Pts',(85.966875037897,16.7151551608915,-1.28752411788782));
#31606=CARTESIAN_POINT('Ctrl Pts',(86.2073738077064,16.0171614768628,4.90467811860692));
#31607=CARTESIAN_POINT('Ctrl Pts',(86.447677494623,13.1077224596251,10.4085994658324));
#31608=CARTESIAN_POINT('Ctrl Pts',(86.6877865663515,8.39163183364423,14.4674371565703));
#31609=CARTESIAN_POINT('Ctrl Pts',(86.9277014259927,2.52521683523347,16.5174726601838));
#31610=CARTESIAN_POINT('Ctrl Pts',(87.2073764041283,-4.71846893122861,16.2531082314488));
#31611=CARTESIAN_POINT('Ctrl Pts',(87.5266824785365,-12.119252917514,12.1679209131024));
#31612=CARTESIAN_POINT('Ctrl Pts',(87.8854707031164,-16.7142851347075,3.84758826535438));
#31613=CARTESIAN_POINT('Ctrl Pts',(88.2438268345246,-16.1808605256974,-5.62684461281575));
#31614=CARTESIAN_POINT('Ctrl Pts',(88.6017596804731,-10.6935017851311,-13.3572996474587));
#31615=CARTESIAN_POINT('Ctrl Pts',(88.9592581284196,-1.94684933313455,-16.9793506731735));
#31616=CARTESIAN_POINT('Ctrl Pts',(89.3163558666232,7.37927353005637,-15.3920445435929));
#31617=CARTESIAN_POINT('Ctrl Pts',(89.6135475815425,13.2414270899268,-10.148282449374));
#31618=CARTESIAN_POINT('Ctrl Pts',(89.8511629514236,15.7308559147538,-4.55632603911814));
#31619=CARTESIAN_POINT('Ctrl Pts',(89.9698142754425,16.1550130455499,-1.57126098134776));
#31620=CARTESIAN_POINT('Ctrl Pts',(90.029242413098,16.157866761838,-0.0321567193703245));
#31621=CARTESIAN_POINT('Ctrl Pts',(68.6597607285732,17.4006280941266,0.00785707557859578));
#31622=CARTESIAN_POINT('Ctrl Pts',(68.7235009699529,17.3975673122243,1.65863870299843));
#31623=CARTESIAN_POINT('Ctrl Pts',(68.8514963705168,16.9400695695691,4.87883884057858));
#31624=CARTESIAN_POINT('Ctrl Pts',(69.1069562397825,14.262686949915,10.8906064157376));
#31625=CARTESIAN_POINT('Ctrl Pts',(69.4266395295462,7.95798755464706,16.5315448855194));
#31626=CARTESIAN_POINT('Ctrl Pts',(69.8101364767553,-2.05974367394959,18.2332011185647));
#31627=CARTESIAN_POINT('Ctrl Pts',(70.1937597880174,-11.4432175552833,14.3466336126088));
#31628=CARTESIAN_POINT('Ctrl Pts',(70.5773880629489,-17.3260775571641,6.0584389009168));
#31629=CARTESIAN_POINT('Ctrl Pts',(70.8971087240495,-17.7947199866996,-2.39254166927833));
#31630=CARTESIAN_POINT('Ctrl Pts',(71.1529016677111,-15.441149366048,-8.53590454680965));
#31631=CARTESIAN_POINT('Ctrl Pts',(71.3447498253948,-12.4775139902205,-12.4777911778366));
#31632=CARTESIAN_POINT('Ctrl Pts',(71.5365993719199,-8.53482928977716,-15.4433197010116));
#31633=CARTESIAN_POINT('Ctrl Pts',(71.7497680377377,-3.41478972728435,-17.3993154029907));
#31634=CARTESIAN_POINT('Ctrl Pts',(71.9842483873757,2.65613898428773,-17.6275734717924));
#31635=CARTESIAN_POINT('Ctrl Pts',(72.2400436052835,8.91240965773181,-15.4378542921431));
#31636=CARTESIAN_POINT('Ctrl Pts',(72.4958333516622,13.9350486173369,-11.1151391614399));
#31637=CARTESIAN_POINT('Ctrl Pts',(72.7516190270194,17.0343485207352,-5.2557825150929));
#31638=CARTESIAN_POINT('Ctrl Pts',(73.0073922590926,17.7722806554582,1.32842090373711));
#31639=CARTESIAN_POINT('Ctrl Pts',(73.3057778782715,15.7784440622631,8.80031303306672));
#31640=CARTESIAN_POINT('Ctrl Pts',(73.6467483653377,9.76765350955319,15.5355999090755));
#31641=CARTESIAN_POINT('Ctrl Pts',(74.0303001928062,0.00324086649956546,
18.3469216573022));
#31642=CARTESIAN_POINT('Ctrl Pts',(74.4137917659782,-9.75515672015961,15.5354418730925));
#31643=CARTESIAN_POINT('Ctrl Pts',(74.7972167116253,-16.5219402379097,7.9627758146546));
#31644=CARTESIAN_POINT('Ctrl Pts',(75.1805634519762,-18.2228041626385,-2.04597779745445));
#31645=CARTESIAN_POINT('Ctrl Pts',(75.5638233687855,-14.3362306118562,-11.4255797117487));
#31646=CARTESIAN_POINT('Ctrl Pts',(75.9469859200462,-6.0636041500258,-17.293973869085));
#31647=CARTESIAN_POINT('Ctrl Pts',(76.3442286759065,4.45035809519592,-17.8921316341132));
#31648=CARTESIAN_POINT('Ctrl Pts',(76.6420630145241,11.2847744272317,-13.8265238405078));
#31649=CARTESIAN_POINT('Ctrl Pts',(76.8973083073728,15.2743398861069,-8.67734593552654));
#31650=CARTESIAN_POINT('Ctrl Pts',(77.0957897594511,17.3348436194496,-3.96875396903001));
#31651=CARTESIAN_POINT('Ctrl Pts',(77.3509344220687,17.5809444731262,2.63986365468201));
#31652=CARTESIAN_POINT('Ctrl Pts',(77.6060046004046,15.3984975693097,8.87656313529381));
#31653=CARTESIAN_POINT('Ctrl Pts',(77.8610143191004,11.0879602445291,13.8853489397089));
#31654=CARTESIAN_POINT('Ctrl Pts',(78.1159555466501,5.24871190651801,16.9710023515976));
#31655=CARTESIAN_POINT('Ctrl Pts',(78.3708228158246,-1.31537487006328,17.7115205686433));
#31656=CARTESIAN_POINT('Ctrl Pts',(78.6256256627463,-7.68805341091284,16.000075751367));
#31657=CARTESIAN_POINT('Ctrl Pts',(78.9086472803925,-13.5973264027015,11.6486643509849));
#31658=CARTESIAN_POINT('Ctrl Pts',(79.1632815997527,-16.7899751467946,5.77830465705051));
#31659=CARTESIAN_POINT('Ctrl Pts',(79.4602587190341,-17.7376470533284,-1.78688963502401));
#31660=CARTESIAN_POINT('Ctrl Pts',(79.7712540029704,-15.4679962299785,-9.69759166027641));
#31661=CARTESIAN_POINT('Ctrl Pts',(80.1527404854897,-7.92824878930432,-16.4318552784184));
#31662=CARTESIAN_POINT('Ctrl Pts',(80.5340186637714,2.02466878417038,-18.1214851807052));
#31663=CARTESIAN_POINT('Ctrl Pts',(80.9150837007837,11.3496854121677,-14.2592766110511));
#31664=CARTESIAN_POINT('Ctrl Pts',(81.2959255170471,17.1852011053556,-6.03175011440449));
#31665=CARTESIAN_POINT('Ctrl Pts',(81.6765347527869,17.7497716308165,4.03117053838598));
#31666=CARTESIAN_POINT('Ctrl Pts',(82.0569046689732,12.8757070820106,12.8510081252502));
#31667=CARTESIAN_POINT('Ctrl Pts',(82.3947862972429,5.04321613190222,17.1718637553676));
#31668=CARTESIAN_POINT('Ctrl Pts',(82.6902738480198,-2.61005988977363,17.4502374567792));
#31669=CARTESIAN_POINT('Ctrl Pts',(82.9434300076959,-8.80025952764612,15.2862649770185));
#31670=CARTESIAN_POINT('Ctrl Pts',(83.1964687178264,-13.7695371664239,11.0080918574343));
#31671=CARTESIAN_POINT('Ctrl Pts',(83.4493880807088,-16.8327170478229,5.21547004081706));
#31672=CARTESIAN_POINT('Ctrl Pts',(83.7021843180637,-17.5641109077076,-1.29378561473781));
#31673=CARTESIAN_POINT('Ctrl Pts',(83.9548528665527,-15.8697255170729,-7.61700457494452));
#31674=CARTESIAN_POINT('Ctrl Pts',(84.2073923691056,-11.9837143457694,-12.8815110092968));
#31675=CARTESIAN_POINT('Ctrl Pts',(84.4598079448926,-6.44679302894026,-16.3617271312645));
#31676=CARTESIAN_POINT('Ctrl Pts',(84.7120847855581,-0.0237395979090416,
-17.5760510646781));
#31677=CARTESIAN_POINT('Ctrl Pts',(84.9642303272761,6.39538656732633,-16.3613398560058));
#31678=CARTESIAN_POINT('Ctrl Pts',(85.2162395408117,11.9238107247879,-12.886977573222));
#31679=CARTESIAN_POINT('Ctrl Pts',(85.4681084387409,15.7994707310197,-7.63609786493631));
#31680=CARTESIAN_POINT('Ctrl Pts',(85.719842902167,17.486012423623,-1.33577274741051));
#31681=CARTESIAN_POINT('Ctrl Pts',(85.9714309934085,16.7559602965917,5.14206670856116));
#31682=CARTESIAN_POINT('Ctrl Pts',(86.2228753368623,13.7117014917251,10.9012971452895));
#31683=CARTESIAN_POINT('Ctrl Pts',(86.4741737949277,8.77584705906915,15.1494265813195));
#31684=CARTESIAN_POINT('Ctrl Pts',(86.7253242351102,2.63465796664165,17.2956018092232));
#31685=CARTESIAN_POINT('Ctrl Pts',(87.0181593012597,-4.94995751639123,17.0189226482735));
#31686=CARTESIAN_POINT('Ctrl Pts',(87.3525707654822,-12.7010842904221,12.7407348698173));
#31687=CARTESIAN_POINT('Ctrl Pts',(87.728436564811,-17.5152394101686,4.0243596939246));
#31688=CARTESIAN_POINT('Ctrl Pts',(88.1039527740728,-16.9565472756951,-5.90364377027598));
#31689=CARTESIAN_POINT('Ctrl Pts',(88.4791004609346,-11.2053993769732,-14.006553928488));
#31690=CARTESIAN_POINT('Ctrl Pts',(88.8539049876026,-2.035744278159,-17.8033917672818));
#31691=CARTESIAN_POINT('Ctrl Pts',(89.2282904122505,7.74277152007772,-16.1403772233317));
#31692=CARTESIAN_POINT('Ctrl Pts',(89.5400581478773,13.8914564051538,-10.6388851155824));
#31693=CARTESIAN_POINT('Ctrl Pts',(89.7891264886643,16.5013623504881,-4.77745809816874));
#31694=CARTESIAN_POINT('Ctrl Pts',(89.9137512217624,16.946855069725,-1.64209065688647));
#31695=CARTESIAN_POINT('Ctrl Pts',(89.97593701968,16.9498412077971,-0.0315669153498612));
#31696=CARTESIAN_POINT('Ctrl Pts',(68.014332389863,16.9368226517689,0.0319184960226097));
#31697=CARTESIAN_POINT('Ctrl Pts',(68.0764705480552,16.9338388012858,1.64120844668688));
#31698=CARTESIAN_POINT('Ctrl Pts',(68.2009984722761,16.4886744022683,4.77406298181688));
#31699=CARTESIAN_POINT('Ctrl Pts',(68.4498749428734,13.8807131815627,10.6308858370252));
#31700=CARTESIAN_POINT('Ctrl Pts',(68.761416689418,7.73692033746066,16.128273198334));
#31701=CARTESIAN_POINT('Ctrl Pts',(69.1355280034991,-2.03476959494914,17.7898195120724));
#31702=CARTESIAN_POINT('Ctrl Pts',(69.5100668032795,-11.1962298165234,13.9962376482653));
#31703=CARTESIAN_POINT('Ctrl Pts',(69.8849504935975,-16.945783170327,5.89821129851622));
#31704=CARTESIAN_POINT('Ctrl Pts',(70.1976715900557,-17.4051344806488,-2.36731702515499));
#31705=CARTESIAN_POINT('Ctrl Pts',(70.4480172764557,-15.101928416316,-8.3797986420383));
#31706=CARTESIAN_POINT('Ctrl Pts',(70.6358677465942,-12.2002491246392,-12.2395111621439));
#31707=CARTESIAN_POINT('Ctrl Pts',(70.8238060359331,-8.33813940883176,-15.1446030697862));
#31708=CARTESIAN_POINT('Ctrl Pts',(71.0327237000049,-3.3204037438702,-17.0616804506108));
#31709=CARTESIAN_POINT('Ctrl Pts',(71.2626597523326,2.63261163312919,-17.2858315776882));
#31710=CARTESIAN_POINT('Ctrl Pts',(71.5136511052112,8.7712694878663,-15.1376581309978));
#31711=CARTESIAN_POINT('Ctrl Pts',(71.7647927622528,13.7027463103588,-10.8939740892587));
#31712=CARTESIAN_POINT('Ctrl Pts',(72.0160805068755,16.7477786072646,-5.13797793175056));
#31713=CARTESIAN_POINT('Ctrl Pts',(72.2675155482385,17.4736046987134,1.33432392506951));
#31714=CARTESIAN_POINT('Ctrl Pts',(72.5610257212911,15.5128311991003,8.68399749862113));
#31715=CARTESIAN_POINT('Ctrl Pts',(72.8967121588295,9.59650585111651,15.3152930648782));
#31716=CARTESIAN_POINT('Ctrl Pts',(73.274669438999,-0.0246868277003993,
18.0868136163285));
#31717=CARTESIAN_POINT('Ctrl Pts',(73.6529358009447,-9.65000244600368,15.315138165857));
#31718=CARTESIAN_POINT('Ctrl Pts',(74.0315016957638,-16.331744326295,7.8397084676337));
#31719=CARTESIAN_POINT('Ctrl Pts',(74.4103614589508,-18.0139710668216,-2.05116003639906));
#31720=CARTESIAN_POINT('Ctrl Pts',(74.7895076049163,-14.170564539168,-11.3301737685776));
#31721=CARTESIAN_POINT('Ctrl Pts',(75.1689333581195,-5.97980433672152,-17.1421185404384));
#31722=CARTESIAN_POINT('Ctrl Pts',(75.5626937216784,4.44136041994808,-17.7365097499734));
#31723=CARTESIAN_POINT('Ctrl Pts',(75.8582312621752,11.2233892267941,-13.7036013137413));
#31724=CARTESIAN_POINT('Ctrl Pts',(76.1116496313081,15.1844323227741,-8.59128840354336));
#31725=CARTESIAN_POINT('Ctrl Pts',(76.3088229628224,17.2314721741726,-3.91415213897931));
#31726=CARTESIAN_POINT('Ctrl Pts',(76.5624281235002,17.4764311383519,2.65449037292804));
#31727=CARTESIAN_POINT('Ctrl Pts',(76.816152542962,15.3060174966826,8.85808296957702));
#31728=CARTESIAN_POINT('Ctrl Pts',(77.0699772467878,11.0159391984402,13.8436381261701));
#31729=CARTESIAN_POINT('Ctrl Pts',(77.3239049175782,5.20035674827198,16.9173023230172));
#31730=CARTESIAN_POINT('Ctrl Pts',(77.577936234861,-1.34181378896731,17.6557574765637));
#31731=CARTESIAN_POINT('Ctrl Pts',(77.8320552996849,-7.69737922244923,15.9493639766937));
#31732=CARTESIAN_POINT('Ctrl Pts',(78.1145243916325,-13.5951231236606,11.6070912487124));
#31733=CARTESIAN_POINT('Ctrl Pts',(78.3688471472273,-16.7844178817442,5.74438589068073));
#31734=CARTESIAN_POINT('Ctrl Pts',(78.6656608116319,-17.7318026091762,-1.81641343765658));
#31735=CARTESIAN_POINT('Ctrl Pts',(78.9767385896377,-15.462822425123,-9.72895758703099));
#31736=CARTESIAN_POINT('Ctrl Pts',(79.3586932597966,-7.91515306456073,-16.4722820318529));
#31737=CARTESIAN_POINT('Ctrl Pts',(79.7408288150502,2.05935680779579,-18.1670862463568));
#31738=CARTESIAN_POINT('Ctrl Pts',(80.1231324309674,11.4147636910949,-14.2938551204881));
#31739=CARTESIAN_POINT('Ctrl Pts',(80.5055971190963,17.2760338856779,-6.03251997755934));
#31740=CARTESIAN_POINT('Ctrl Pts',(80.8882139858091,17.844936685304,4.08285450666647));
#31741=CARTESIAN_POINT('Ctrl Pts',(81.2709714329646,12.9417717016896,12.9583263956821));
#31742=CARTESIAN_POINT('Ctrl Pts',(81.6113241079054,5.05304097073616,17.3115655713565));
#31743=CARTESIAN_POINT('Ctrl Pts',(81.9092036538918,-2.66196224769219,17.5926673075212));
#31744=CARTESIAN_POINT('Ctrl Pts',(82.1645848689637,-8.90638889298226,15.4101212359073));
#31745=CARTESIAN_POINT('Ctrl Pts',(82.4200136325472,-13.9227166542397,11.0920226111291));
#31746=CARTESIAN_POINT('Ctrl Pts',(82.6754866039489,-17.0170240494153,5.24127019003033));
#31747=CARTESIAN_POINT('Ctrl Pts',(82.9310030857056,-17.756717250709,-1.33778819487169));
#31748=CARTESIAN_POINT('Ctrl Pts',(83.1865644655235,-16.0433394548369,-7.73323614893282));
#31749=CARTESIAN_POINT('Ctrl Pts',(83.4421661736319,-12.1107655448105,-13.0615834286996));
#31750=CARTESIAN_POINT('Ctrl Pts',(83.6977931804047,-6.50370995420041,-16.586309544005));
#31751=CARTESIAN_POINT('Ctrl Pts',(83.9534640397682,0.00531481089540298,
-17.8173430226054));
#31752=CARTESIAN_POINT('Ctrl Pts',(84.2091594317815,6.5146243017338,-16.5859416183189));
#31753=CARTESIAN_POINT('Ctrl Pts',(84.4648814125953,12.12450727094,-13.0609202293272));
#31754=CARTESIAN_POINT('Ctrl Pts',(84.7206310049753,16.0599935964609,-7.72964432252528));
#31755=CARTESIAN_POINT('Ctrl Pts',(84.9763905740002,17.7738878064829,-1.32882848634198));
#31756=CARTESIAN_POINT('Ctrl Pts',(85.2321758096326,17.03207406858,5.25685256337923));
#31757=CARTESIAN_POINT('Ctrl Pts',(85.4879751575384,13.9355754035496,11.1157872024267));
#31758=CARTESIAN_POINT('Ctrl Pts',(85.7437858116849,8.91155809052332,15.4403568542271));
#31759=CARTESIAN_POINT('Ctrl Pts',(85.9996060974355,2.65654793570823,17.6267315370253));
#31760=CARTESIAN_POINT('Ctrl Pts',(86.2980666948127,-5.07351735129217,17.3452336162104));
#31761=CARTESIAN_POINT('Ctrl Pts',(86.6391833189476,-12.9801532360575,12.9825944194009));
#31762=CARTESIAN_POINT('Ctrl Pts',(87.0229268046549,-17.8961913498233,4.08451505234094));
#31763=CARTESIAN_POINT('Ctrl Pts',(87.4066687860505,-17.3265839015146,-6.0604305607405));
#31764=CARTESIAN_POINT('Ctrl Pts',(87.7903709222829,-11.4455386605879,-14.348712512324));
#31765=CARTESIAN_POINT('Ctrl Pts',(88.1740825929623,-2.05902204053203,-18.2363604026539));
#31766=CARTESIAN_POINT('Ctrl Pts',(88.5576667221726,7.96004300481042,-16.5342363554814));
#31767=CARTESIAN_POINT('Ctrl Pts',(88.8774482190082,14.2667445785016,-10.8921034944438));
#31768=CARTESIAN_POINT('Ctrl Pts',(89.1329596343274,16.9446486652469,-4.87923821628262));
#31769=CARTESIAN_POINT('Ctrl Pts',(89.2609907780456,17.4024388597611,-1.65829899794939));
#31770=CARTESIAN_POINT('Ctrl Pts',(89.3247406611467,17.4055001046014,-0.0072676741977367));
#31771=CARTESIAN_POINT('Ctrl Pts',(67.9785110845474,16.1431896342132,0.0318301264118968));
#31772=CARTESIAN_POINT('Ctrl Pts',(68.0378858846227,16.1403384791252,1.569553030724));
#31773=CARTESIAN_POINT('Ctrl Pts',(68.1564254451454,15.7165770004678,4.55178190463174));
#31774=CARTESIAN_POINT('Ctrl Pts',(68.3938219334874,13.2293798077654,10.1385336217139));
#31775=CARTESIAN_POINT('Ctrl Pts',(68.6907420120926,7.37292663615509,15.3774902252066));
#31776=CARTESIAN_POINT('Ctrl Pts',(69.0475082724276,-1.94493333057598,16.9631236785857));
#31777=CARTESIAN_POINT('Ctrl Pts',(69.4046728281513,-10.6819468555142,13.3449418751655));
#31778=CARTESIAN_POINT('Ctrl Pts',(69.7622677199762,-16.1665520224338,5.62093383043492));
#31779=CARTESIAN_POINT('Ctrl Pts',(70.0606157014478,-16.60504542502,-2.26502246803787));
#31780=CARTESIAN_POINT('Ctrl Pts',(70.2995058763236,-14.4073009182687,-8.00238558857723));
#31781=CARTESIAN_POINT('Ctrl Pts',(70.4787806828198,-11.6380989564286,-11.6859690320109));
#31782=CARTESIAN_POINT('Ctrl Pts',(70.6581631675788,-7.95182529872869,-14.4588656285554));
#31783=CARTESIAN_POINT('Ctrl Pts',(70.8575964721588,-3.16186856987872,-16.2889865245856));
#31784=CARTESIAN_POINT('Ctrl Pts',(71.0771282073065,2.52182904090697,-16.5031150354075));
#31785=CARTESIAN_POINT('Ctrl Pts',(71.3168096314304,8.38398534374628,-14.4518485098465));
#31786=CARTESIAN_POINT('Ctrl Pts',(71.5566843359071,13.0943431381348,-10.3985989843744));
#31787=CARTESIAN_POINT('Ctrl Pts',(71.7967518576259,16.0035661257044,-4.89963928653314));
#31788=CARTESIAN_POINT('Ctrl Pts',(72.0370139613808,16.6972678826331,1.28510323855206));
#31789=CARTESIAN_POINT('Ctrl Pts',(72.3175466529949,14.8233549849365,8.30992155597743));
#31790=CARTESIAN_POINT('Ctrl Pts',(72.6384820627477,9.16722602236474,14.6502440480075));
#31791=CARTESIAN_POINT('Ctrl Pts',(72.9999735466316,-0.034818267257906,
17.301604261126));
#31792=CARTESIAN_POINT('Ctrl Pts',(73.3619064145069,-9.24486652526365,14.6501004295558));
#31793=CARTESIAN_POINT('Ctrl Pts',(73.7242810319573,-15.641416905871,7.49465763351948));
#31794=CARTESIAN_POINT('Ctrl Pts',(74.0870981624789,-17.2530825064288,-1.97749200747249));
#31795=CARTESIAN_POINT('Ctrl Pts',(74.4503580843669,-13.571256654549,-10.8681906954034));
#31796=CARTESIAN_POINT('Ctrl Pts',(74.8140609279404,-5.72011949551101,-16.440006102462));
#31797=CARTESIAN_POINT('Ctrl Pts',(75.1916935457088,4.27441446084024,-17.0108569349597));
#31798=CARTESIAN_POINT('Ctrl Pts',(75.4752811028074,10.7827639267889,-13.1414831702565));
#31799=CARTESIAN_POINT('Ctrl Pts',(75.7185548673632,14.5853175807895,-8.23381412747197));
#31800=CARTESIAN_POINT('Ctrl Pts',(75.907867413484,16.5509807384611,-3.74306843918247));
#31801=CARTESIAN_POINT('Ctrl Pts',(76.1514680483462,16.7865607653339,2.56649192426096));
#31802=CARTESIAN_POINT('Ctrl Pts',(76.3952622907919,14.7012372504299,8.52757133361821));
#31803=CARTESIAN_POINT('Ctrl Pts',(76.6392530801337,10.577484401339,13.3202749579265));
#31804=CARTESIAN_POINT('Ctrl Pts',(76.883439294177,4.98496285112783,16.2762918787137));
#31805=CARTESIAN_POINT('Ctrl Pts',(77.1278192754108,-1.30884007541534,16.9869922345478));
#31806=CARTESIAN_POINT('Ctrl Pts',(77.3723966666688,-7.42591453522203,15.3448479448429));
#31807=CARTESIAN_POINT('Ctrl Pts',(77.6443621377783,-13.1046908653612,11.1641662681244));
#31808=CARTESIAN_POINT('Ctrl Pts',(77.8893591794915,-16.1774889930477,5.51654176568881));
#31809=CARTESIAN_POINT('Ctrl Pts',(78.1754139623,-17.0906981982566,-1.7703111468904));
#31810=CARTESIAN_POINT('Ctrl Pts',(78.4753399201003,-14.9036520345214,-9.39974734360126));
#31811=CARTESIAN_POINT('Ctrl Pts',(78.8438648610653,-7.62177045923067,-15.9069310852974));
#31812=CARTESIAN_POINT('Ctrl Pts',(79.2128171384923,2.00889070682572,-17.5442570054289));
#31813=CARTESIAN_POINT('Ctrl Pts',(79.5821956018624,11.0487422668153,-13.8027572119352));
#31814=CARTESIAN_POINT('Ctrl Pts',(79.9519969108647,16.7170242555458,-5.81521116669086));
#31815=CARTESIAN_POINT('Ctrl Pts',(80.3222172565172,17.2685968035139,3.97281760370441));
#31816=CARTESIAN_POINT('Ctrl Pts',(80.6928547291618,12.5214581392903,12.5681324652044));
#31817=CARTESIAN_POINT('Ctrl Pts',(81.0226741018505,4.87690503480926,16.7877757436989));
#31818=CARTESIAN_POINT('Ctrl Pts',(81.3115367942124,-2.60480142711277,17.0607827981659));
#31819=CARTESIAN_POINT('Ctrl Pts',(81.5593120712615,-8.66362909419818,14.943484187758));
#31820=CARTESIAN_POINT('Ctrl Pts',(81.8072681247254,-13.5335698559155,10.7518132776484));
#31821=CARTESIAN_POINT('Ctrl Pts',(82.0554037496435,-16.5394462539352,5.06910782949574));
#31822=CARTESIAN_POINT('Ctrl Pts',(82.3037169758971,-17.2586053337516,-1.32463910810424));
#31823=CARTESIAN_POINT('Ctrl Pts',(82.5522036597656,-15.5929741482425,-7.54339860049728));
#31824=CARTESIAN_POINT('Ctrl Pts',(82.8008637977723,-11.7672571729509,-12.7274796411849));
#31825=CARTESIAN_POINT('Ctrl Pts',(83.0497030317913,-6.30918200043825,-16.1590093563318));
#31826=CARTESIAN_POINT('Ctrl Pts',(83.2987071571274,0.030423146966114,-17.3583257425452));
#31827=CARTESIAN_POINT('Ctrl Pts',(83.5478845422533,6.37414250483962,-16.1586487421449));
#31828=CARTESIAN_POINT('Ctrl Pts',(83.7972310681378,11.8445640374261,-12.7216220956902));
#31829=CARTESIAN_POINT('Ctrl Pts',(84.0467422766515,15.6845723764937,-7.52032796424948));
#31830=CARTESIAN_POINT('Ctrl Pts',(84.2964270384935,17.3581049205115,-1.27147299465656));
#31831=CARTESIAN_POINT('Ctrl Pts',(84.5462707233275,16.6338652686637,5.16156858897617));
#31832=CARTESIAN_POINT('Ctrl Pts',(84.7962779718032,13.6076521978334,10.8882602246653));
#31833=CARTESIAN_POINT('Ctrl Pts',(85.0464468759817,8.69445958734289,15.1178971036121));
#31834=CARTESIAN_POINT('Ctrl Pts',(85.2967753376485,2.57355346225438,17.2577590241979));
#31835=CARTESIAN_POINT('Ctrl Pts',(85.5890114258584,-4.99555256481923,16.982557096495));
#31836=CARTESIAN_POINT('Ctrl Pts',(85.9232482985609,-12.7437747387513,12.7085701664197));
#31837=CARTESIAN_POINT('Ctrl Pts',(86.2996124177631,-17.5666805845105,3.98182266229514));
#31838=CARTESIAN_POINT('Ctrl Pts',(86.6763192307827,-17.0088110427856,-5.97792722908082));
#31839=CARTESIAN_POINT('Ctrl Pts',(87.0533497486091,-11.2308662184509,-14.1231298760299));
#31840=CARTESIAN_POINT('Ctrl Pts',(87.4307284834426,-1.99915391505435,-17.9484835097794));
#31841=CARTESIAN_POINT('Ctrl Pts',(87.8083766725088,7.86516832083256,-16.2735894236369));
#31842=CARTESIAN_POINT('Ctrl Pts',(88.1234384738727,14.0802153362982,-10.7153937271007));
#31843=CARTESIAN_POINT('Ctrl Pts',(88.3754809575467,16.721833883369,-4.78406246384038));
#31844=CARTESIAN_POINT('Ctrl Pts',(88.50174380989,17.173221591803,-1.60746207645487));
#31845=CARTESIAN_POINT('Ctrl Pts',(88.5646803557127,17.1762437805005,0.0225049683035558));
#31846=CARTESIAN_POINT('Ctrl Pts',(68.5732254931795,15.6164607114294,0.00789028987868486));
#31847=CARTESIAN_POINT('Ctrl Pts',(68.6307543287869,15.613698198846,1.49780533901795));
#31848=CARTESIAN_POINT('Ctrl Pts',(68.7452888582432,15.2043138900613,4.37940633245871));
#31849=CARTESIAN_POINT('Ctrl Pts',(68.9749441538233,12.7983847167288,9.78409544822882));
#31850=CARTESIAN_POINT('Ctrl Pts',(69.2617618377016,7.13956805019415,14.844065966187));
#31851=CARTESIAN_POINT('Ctrl Pts',(69.6062737406281,-1.85807669057325,16.3750371655707));
#31852=CARTESIAN_POINT('Ctrl Pts',(69.9508498703511,-10.2875139219393,12.88262556287));
#31853=CARTESIAN_POINT('Ctrl Pts',(70.2956244517574,-15.5748451070192,5.43501177969178));
#31854=CARTESIAN_POINT('Ctrl Pts',(70.5830503952178,-15.9965254225249,-2.16296862263973));
#31855=CARTESIAN_POINT('Ctrl Pts',(70.8130992683074,-13.8799527336818,-7.68799620388367));
#31856=CARTESIAN_POINT('Ctrl Pts',(70.9856768912645,-11.2140225776427,-11.2340383430839));
#31857=CARTESIAN_POINT('Ctrl Pts',(71.1583013094849,-7.66647800099633,-13.9024562467762));
#31858=CARTESIAN_POINT('Ctrl Pts',(71.3501585789615,-3.05831667813383,-15.6630039154817));
#31859=CARTESIAN_POINT('Ctrl Pts',(71.5612650719921,2.40745597291645,-15.8686977749241));
#31860=CARTESIAN_POINT('Ctrl Pts',(71.79165252113,8.04240760846629,-13.896683013927));
#31861=CARTESIAN_POINT('Ctrl Pts',(72.0221311730022,12.5682094894439,-10.0018632134027));
#31862=CARTESIAN_POINT('Ctrl Pts',(72.2527081604281,15.3622886786739,-4.72008117234861));
#31863=CARTESIAN_POINT('Ctrl Pts',(72.4833799691409,16.0280497202866,1.21795506808586));
#31864=CARTESIAN_POINT('Ctrl Pts',(72.7526121354263,14.229337115007,7.95988872480797));
#31865=CARTESIAN_POINT('Ctrl Pts',(73.0604623958875,8.80304371259818,14.0415174266253));
#31866=CARTESIAN_POINT('Ctrl Pts',(73.4070369783453,-0.0197241229505961,
16.5828396759277));
#31867=CARTESIAN_POINT('Ctrl Pts',(73.7538537051601,-8.84521045017838,14.0413090669527));
#31868=CARTESIAN_POINT('Ctrl Pts',(74.1009242982494,-14.9712897991147,7.18743784651643));
#31869=CARTESIAN_POINT('Ctrl Pts',(74.4482544704108,-16.5135836921132,-1.88073950663067));
#31870=CARTESIAN_POINT('Ctrl Pts',(74.7958523761652,-12.9898701817829,-10.3880820430838));
#31871=CARTESIAN_POINT('Ctrl Pts',(75.1437249277752,-5.479968520301,-15.7170578917619));
#31872=CARTESIAN_POINT('Ctrl Pts',(75.5047745491095,4.07591305069949,-16.2622748769602));
#31873=CARTESIAN_POINT('Ctrl Pts',(75.775799333639,10.2958255109986,-12.5638294058234));
#31874=CARTESIAN_POINT('Ctrl Pts',(76.0082498170727,13.9291885586121,-7.8745029993023));
#31875=CARTESIAN_POINT('Ctrl Pts',(76.1891039657334,15.8069677171505,-3.58426467255911));
#31876=CARTESIAN_POINT('Ctrl Pts',(76.4217770053772,16.0318674553836,2.44227285229655));
#31877=CARTESIAN_POINT('Ctrl Pts',(76.6545783736397,14.040403264277,8.13460446657749));
#31878=CARTESIAN_POINT('Ctrl Pts',(76.8875232761733,10.1032200457297,12.7102945419314));
#31879=CARTESIAN_POINT('Ctrl Pts',(77.1206092391391,4.76480431332326,15.5318472041218));
#31880=CARTESIAN_POINT('Ctrl Pts',(77.3538369474926,-1.2418588919811,16.2099981882822));
#31881=CARTESIAN_POINT('Ctrl Pts',(77.5872162447358,-7.07885707968089,14.6429296330323));
#31882=CARTESIAN_POINT('Ctrl Pts',(77.846685398312,-12.4966715102306,10.6542004249985));
#31883=CARTESIAN_POINT('Ctrl Pts',(78.0803862302803,-15.4276682037717,5.26688438574245));
#31884=CARTESIAN_POINT('Ctrl Pts',(78.3532145233418,-16.2985957883637,-1.68306604566752));
#31885=CARTESIAN_POINT('Ctrl Pts',(78.639230520238,-14.2127530389122,-8.95864314282349));
#31886=CARTESIAN_POINT('Ctrl Pts',(78.9906062755114,-7.26956674749928,-15.1628401104227));
#31887=CARTESIAN_POINT('Ctrl Pts',(79.3423379425772,1.91162644513308,-16.7235371996257));
#31888=CARTESIAN_POINT('Ctrl Pts',(79.6944332129699,10.5284119075426,-13.1569449089522));
#31889=CARTESIAN_POINT('Ctrl Pts',(80.0468964689781,15.9307968428758,-5.54383713737964));
#31890=CARTESIAN_POINT('Ctrl Pts',(80.3997335729651,16.4563471991834,3.7845448884978));
#31891=CARTESIAN_POINT('Ctrl Pts',(80.7529499471889,11.9322974734141,11.9757512534284));
#31892=CARTESIAN_POINT('Ctrl Pts',(81.0672605152526,4.64727666760693,15.9968648754117));
#31893=CARTESIAN_POINT('Ctrl Pts',(81.3425355553074,-2.48245353398034,16.2570098744713));
#31894=CARTESIAN_POINT('Ctrl Pts',(81.578659307521,-8.25629043460913,14.2392789277651));
#31895=CARTESIAN_POINT('Ctrl Pts',(81.8149585891481,-12.8972496915939,10.2447011996574));
#31896=CARTESIAN_POINT('Ctrl Pts',(82.0514351845093,-15.7618455262871,4.82905942687374));
#31897=CARTESIAN_POINT('Ctrl Pts',(82.2880894843119,-16.4472559956533,-1.26442742198006));
#31898=CARTESIAN_POINT('Ctrl Pts',(82.5249231812786,-14.859753523671,-7.19146106306312));
#31899=CARTESIAN_POINT('Ctrl Pts',(82.7619370618063,-11.2133046829268,-12.1326712627875));
#31900=CARTESIAN_POINT('Ctrl Pts',(82.9991329362443,-6.01067514441112,-15.4036195228323));
#31901=CARTESIAN_POINT('Ctrl Pts',(83.2365115257908,0.0328026357451166,
-16.5469545639429));
#31902=CARTESIAN_POINT('Ctrl Pts',(83.4740741545337,6.08071192374398,-15.4032396381725));
#31903=CARTESIAN_POINT('Ctrl Pts',(83.7118214220829,11.2965930002099,-12.1262135570267));
#31904=CARTESIAN_POINT('Ctrl Pts',(83.9497552306074,14.9583526864088,-7.166418458723));
#31905=CARTESIAN_POINT('Ctrl Pts',(84.1878744720314,16.5544286075028,-1.20709720700542));
#31906=CARTESIAN_POINT('Ctrl Pts',(84.4261826539153,15.8636982242883,4.92878564118838));
#31907=CARTESIAN_POINT('Ctrl Pts',(84.6646792725393,12.9769490355419,10.3917177919627));
#31908=CARTESIAN_POINT('Ctrl Pts',(84.9033652615053,8.28944183209289,14.4271871126583));
#31909=CARTESIAN_POINT('Ctrl Pts',(85.1422415313731,2.44872748562762,16.4691811951198));
#31910=CARTESIAN_POINT('Ctrl Pts',(85.4211527257243,-4.77508597602963,16.2066560777324));
#31911=CARTESIAN_POINT('Ctrl Pts',(85.7402304059049,-12.1717760149211,12.1269180477954));
#31912=CARTESIAN_POINT('Ctrl Pts',(86.0996256302246,-16.7773770828534,3.79415904445876));
#31913=CARTESIAN_POINT('Ctrl Pts',(86.4594555284599,-16.2449490675834,-5.71927479188544));
#31914=CARTESIAN_POINT('Ctrl Pts',(86.8197255804431,-10.7244313897633,-13.50198698288));
#31915=CARTESIAN_POINT('Ctrl Pts',(87.1804283172508,-1.90077784239629,-17.1593109571835));
#31916=CARTESIAN_POINT('Ctrl Pts',(87.5415861772252,7.5319100185124,-15.5572454672215));
#31917=CARTESIAN_POINT('Ctrl Pts',(87.8428916470029,13.4767793834455,-10.2428656830246));
#31918=CARTESIAN_POINT('Ctrl Pts',(88.084202234992,16.0056354393952,-4.56413387924517));
#31919=CARTESIAN_POINT('Ctrl Pts',(88.2048947778817,16.4372214891323,-1.52778189497975));
#31920=CARTESIAN_POINT('Ctrl Pts',(88.265253815439,16.4401199068752,0.0354313507669335));
#31921=CARTESIAN_POINT('Ctrl Pts',(69.3554865621267,15.7586009948934,-0.0220509501548168));
#31922=CARTESIAN_POINT('Ctrl Pts',(69.4134811104057,15.7558161189664,1.47992539504222));
#31923=CARTESIAN_POINT('Ctrl Pts',(69.5290493343402,15.3425635750154,4.38734680893652));
#31924=CARTESIAN_POINT('Ctrl Pts',(69.7605748863597,12.916682078002,9.83583944427305));
#31925=CARTESIAN_POINT('Ctrl Pts',(70.0495466337453,7.21496031817409,14.9325634258652));
#31926=CARTESIAN_POINT('Ctrl Pts',(70.3962293867449,-1.83928108127539,16.4716096115821));
#31927=CARTESIAN_POINT('Ctrl Pts',(70.7426082400899,-10.31166028394,12.9599789925058));
#31928=CARTESIAN_POINT('Ctrl Pts',(71.0887904289397,-15.6191617372178,5.48152514440198));
#31929=CARTESIAN_POINT('Ctrl Pts',(71.3770873439344,-16.0409364055185,-2.13882427430054));
#31930=CARTESIAN_POINT('Ctrl Pts',(71.6076152300708,-13.9198137867518,-7.67505850180117));
#31931=CARTESIAN_POINT('Ctrl Pts',(71.7804597344815,-11.2497340227708,-11.2263471634346));
#31932=CARTESIAN_POINT('Ctrl Pts',(71.9532548218948,-7.69870714190467,-13.8971433806351));
#31933=CARTESIAN_POINT('Ctrl Pts',(72.1451937394336,-3.08867215696627,-15.6581893785022));
#31934=CARTESIAN_POINT('Ctrl Pts',(72.356261775191,2.37585195054601,-15.8634589022843));
#31935=CARTESIAN_POINT('Ctrl Pts',(72.5864337561947,8.00512203809534,-13.8929836091311));
#31936=CARTESIAN_POINT('Ctrl Pts',(72.816525322706,12.5229127584701,-10.0046290172406));
#31937=CARTESIAN_POINT('Ctrl Pts',(73.0465358476154,15.309660950597,-4.73576036816845));
#31938=CARTESIAN_POINT('Ctrl Pts',(73.276472152517,15.9729502769563,1.18315283570215));
#31939=CARTESIAN_POINT('Ctrl Pts',(73.5446463126725,14.1808529658398,7.89830187925463));
#31940=CARTESIAN_POINT('Ctrl Pts',(73.851023436174,8.78001534186335,13.9496872794977));
#31941=CARTESIAN_POINT('Ctrl Pts',(74.1955442149099,0.00951954523056671,
16.4744918719307));
#31942=CARTESIAN_POINT('Ctrl Pts',(74.5399278818977,-8.75322061768005,13.949641737885));
#31943=CARTESIAN_POINT('Ctrl Pts',(74.8841816357822,-14.8282967853525,7.15077110646269));
#31944=CARTESIAN_POINT('Ctrl Pts',(75.228316026177,-16.3549723822615,-1.83380979289747));
#31945=CARTESIAN_POINT('Ctrl Pts',(75.5723397010806,-12.8663512055993,-10.2527952448652));
#31946=CARTESIAN_POINT('Ctrl Pts',(75.9162626563545,-5.44121162363188,-15.5199611086518));
#31947=CARTESIAN_POINT('Ctrl Pts',(76.2728291254588,3.99577624336786,-16.0569242553695));
#31948=CARTESIAN_POINT('Ctrl Pts',(76.5401884256857,10.1306890549616,-12.4075975768256));
#31949=CARTESIAN_POINT('Ctrl Pts',(76.7693156308531,13.7120020373686,-7.78532179148715));
#31950=CARTESIAN_POINT('Ctrl Pts',(76.9475149829319,15.5619033942757,-3.55809108490052));
#31951=CARTESIAN_POINT('Ctrl Pts',(77.1765954339299,15.7828857769102,2.37536910232938));
#31952=CARTESIAN_POINT('Ctrl Pts',(77.4056552297485,13.8231696965287,7.97591454512957));
#31953=CARTESIAN_POINT('Ctrl Pts',(77.6346912714932,9.95182205786405,12.4744758684292));
#31954=CARTESIAN_POINT('Ctrl Pts',(77.8637085143845,4.70655604086376,15.2464176389137));
#31955=CARTESIAN_POINT('Ctrl Pts',(78.0927102070453,-1.19116127275504,15.9118920613635));
#31956=CARTESIAN_POINT('Ctrl Pts',(78.321696409481,-6.91812279056631,14.3740271026128));
#31957=CARTESIAN_POINT('Ctrl Pts',(78.5761156945386,-12.2301612837638,10.4626553659842));
#31958=CARTESIAN_POINT('Ctrl Pts',(78.8050826972065,-15.1012059510755,5.18423341933701));
#31959=CARTESIAN_POINT('Ctrl Pts',(79.0722068078515,-15.9537211944819,-1.62036410733684));
#31960=CARTESIAN_POINT('Ctrl Pts',(79.3520505918744,-13.9120232543956,-8.73854028938565));
#31961=CARTESIAN_POINT('Ctrl Pts',(79.6954998806611,-7.12472860195661,-14.8017620279139));
#31962=CARTESIAN_POINT('Ctrl Pts',(80.038964842755,1.8407196869181,-16.3245995393403));
#31963=CARTESIAN_POINT('Ctrl Pts',(80.3824543573656,10.2463570189986,-12.8441193957147));
#31964=CARTESIAN_POINT('Ctrl Pts',(80.7259783705505,15.510715150953,-5.42350262165804));
#31965=CARTESIAN_POINT('Ctrl Pts',(81.0695469282049,16.0213174103418,3.65983970761737));
#31966=CARTESIAN_POINT('Ctrl Pts',(81.4131701287784,11.6191576623806,11.6279814012209));
#31967=CARTESIAN_POINT('Ctrl Pts',(81.7186693781985,4.53794766693765,15.5355013496972));
#31968=CARTESIAN_POINT('Ctrl Pts',(81.9860293495058,-2.38675512585456,15.7877899821334));
#31969=CARTESIAN_POINT('Ctrl Pts',(82.215230127172,-7.99122526150496,13.8289386577737));
#31970=CARTESIAN_POINT('Ctrl Pts',(82.4444696685961,-12.4933309249039,9.95347113038892));
#31971=CARTESIAN_POINT('Ctrl Pts',(82.673750686035,-15.2705152113464,4.70245808038809));
#31972=CARTESIAN_POINT('Ctrl Pts',(82.9030760103164,-15.9344030721451,-1.20235742623294));
#31973=CARTESIAN_POINT('Ctrl Pts',(83.1324471253651,-14.396643605772,-6.9425988949701));
#31974=CARTESIAN_POINT('Ctrl Pts',(83.3618675312114,-10.8667692731275,-11.7253679559343));
#31975=CARTESIAN_POINT('Ctrl Pts',(83.5913426476898,-5.83330998696166,-14.889628493777));
#31976=CARTESIAN_POINT('Ctrl Pts',(83.8208701982859,0.0103976999952868,
-15.9948935423422));
#31977=CARTESIAN_POINT('Ctrl Pts',(84.0504569625436,5.85526780827805,-14.8893117845691));
#31978=CARTESIAN_POINT('Ctrl Pts',(84.2801046886058,10.8933554968448,-11.7236661989334));
#31979=CARTESIAN_POINT('Ctrl Pts',(84.5098145369384,14.4284025727732,-6.93508138626014));
#31980=CARTESIAN_POINT('Ctrl Pts',(84.7395942161118,15.9683236638494,-1.18436897605337));
#31981=CARTESIAN_POINT('Ctrl Pts',(84.9694401440822,15.3018668690941,4.73368770101318));
#31982=CARTESIAN_POINT('Ctrl Pts',(85.1993580490269,12.5186922290628,10.0000809026083));
#31983=CARTESIAN_POINT('Ctrl Pts',(85.4293506363143,8.00167975043132,13.8884351919084));
#31984=CARTESIAN_POINT('Ctrl Pts',(85.6594199151074,2.37613020638112,15.8549524353607));
#31985=CARTESIAN_POINT('Ctrl Pts',(85.9279288353029,-4.57837170569589,15.6019263798431));
#31986=CARTESIAN_POINT('Ctrl Pts',(86.2349268185622,-11.6949474665043,11.6758532799693));
#31987=CARTESIAN_POINT('Ctrl Pts',(86.5804999095392,-16.1227972318607,3.66306032098784));
#31988=CARTESIAN_POINT('Ctrl Pts',(86.9262673138911,-15.6104368586567,-5.47901881528954));
#31989=CARTESIAN_POINT('Ctrl Pts',(87.2722614297209,-10.308000965391,-12.952773643117));
#31990=CARTESIAN_POINT('Ctrl Pts',(87.6184399210169,-1.83881862598979,-16.4630114594182));
#31991=CARTESIAN_POINT('Ctrl Pts',(87.9649223234146,7.2099881294249,-14.9245647492593));
#31992=CARTESIAN_POINT('Ctrl Pts',(88.2537065209088,12.9084970264012,-9.83094298475437));
#31993=CARTESIAN_POINT('Ctrl Pts',(88.4851031381616,15.3329342416512,-4.3853617140389));
#31994=CARTESIAN_POINT('Ctrl Pts',(88.6005976121871,15.745854566904,-1.47969784819705));
#31995=CARTESIAN_POINT('Ctrl Pts',(88.6585631413514,15.7486380492955,0.0215269336002149));
#31996=CARTESIAN_POINT('Ctrl Pts',(69.6070021409208,16.2225732106956,-0.030902239567753));
#31997=CARTESIAN_POINT('Ctrl Pts',(69.6666095923113,16.2197108837808,1.51284600302981));
#31998=CARTESIAN_POINT('Ctrl Pts',(69.7856674073585,15.7940421807546,4.50812319888975));
#31999=CARTESIAN_POINT('Ctrl Pts',(70.0238631486952,13.2979406585872,10.1135870839616));
#32000=CARTESIAN_POINT('Ctrl Pts',(70.3212301672275,7.43083592330514,15.3586300203037));
#32001=CARTESIAN_POINT('Ctrl Pts',(70.6777768910567,-1.88174215475493,16.9404787438039));
#32002=CARTESIAN_POINT('Ctrl Pts',(71.0339167259705,-10.5926919897194,13.3297345456673));
#32003=CARTESIAN_POINT('Ctrl Pts',(71.3897046015357,-16.0471465206019,5.64301645195004));
#32004=CARTESIAN_POINT('Ctrl Pts',(71.6858849274608,-16.4799945267065,-2.18584392000218));
#32005=CARTESIAN_POINT('Ctrl Pts',(71.9226506457541,-14.3013440642795,-7.87192383812878));
#32006=CARTESIAN_POINT('Ctrl Pts',(72.1001347007795,-11.5594963624761,-11.5185330246076));
#32007=CARTESIAN_POINT('Ctrl Pts',(72.2775300867685,-7.91383757171182,-14.2604076269911));
#32008=CARTESIAN_POINT('Ctrl Pts',(72.4745372394819,-3.18199126478013,-16.0678915474459));
#32009=CARTESIAN_POINT('Ctrl Pts',(72.6911206000822,2.42541506478198,-16.278352413953));
#32010=CARTESIAN_POINT('Ctrl Pts',(72.9272379722367,8.20009129902322,-14.2567707145772));
#32011=CARTESIAN_POINT('Ctrl Pts',(73.1632010972874,12.8330823756507,-10.2689825602553));
#32012=CARTESIAN_POINT('Ctrl Pts',(73.3990107185643,15.6899365867221,-4.86715147392478));
#32013=CARTESIAN_POINT('Ctrl Pts',(73.6346690720767,16.3695278473878,1.19911655094387));
#32014=CARTESIAN_POINT('Ctrl Pts',(73.9094295079317,14.5331741821317,8.07916458355286));
#32015=CARTESIAN_POINT('Ctrl Pts',(74.2231998790054,9.00147961852772,14.2762190647474));
#32016=CARTESIAN_POINT('Ctrl Pts',(74.5758598201176,0.0235694186269233,
16.859981462138));
#32017=CARTESIAN_POINT('Ctrl Pts',(74.9281977685756,-8.94137318857348,14.276105227731));
#32018=CARTESIAN_POINT('Ctrl Pts',(75.2802179203447,-15.1529298525304,7.32337194121319));
#32019=CARTESIAN_POINT('Ctrl Pts',(75.6319267377427,-16.7124468093521,-1.85904424112892));
#32020=CARTESIAN_POINT('Ctrl Pts',(75.9833295246471,-13.1483029282851,-10.4582351450381));
#32021=CARTESIAN_POINT('Ctrl Pts',(76.3344329097446,-5.56776703481709,-15.8346725704608));
#32022=CARTESIAN_POINT('Ctrl Pts',(76.6982359590696,4.06068437376695,-16.3816517697198));
#32023=CARTESIAN_POINT('Ctrl Pts',(76.9708544639752,10.3157792069132,-12.6599643611329));
#32024=CARTESIAN_POINT('Ctrl Pts',(77.2043879176041,13.965893382995,-7.94880609169154));
#32025=CARTESIAN_POINT('Ctrl Pts',(77.3859744123835,15.8507322928185,-3.64123533389424));
#32026=CARTESIAN_POINT('Ctrl Pts',(77.6193054202522,16.0755335889672,2.40228153812341));
#32027=CARTESIAN_POINT('Ctrl Pts',(77.8525294367406,14.0799995000416,8.10441349915241));
#32028=CARTESIAN_POINT('Ctrl Pts',(78.0856299239375,10.1398119136579,12.6825221559361));
#32029=CARTESIAN_POINT('Ctrl Pts',(78.3186141911062,4.80368400525854,15.5022129275132));
#32030=CARTESIAN_POINT('Ctrl Pts',(78.5514889552242,-1.19363492880806,16.1786335212657));
#32031=CARTESIAN_POINT('Ctrl Pts',(78.7842389031178,-7.01459644633699,14.6153021683494));
#32032=CARTESIAN_POINT('Ctrl Pts',(79.0427392288324,-12.4115223173748,10.6410404315552));
#32033=CARTESIAN_POINT('Ctrl Pts',(79.2752536639931,-15.3266141779886,5.28072960093371));
#32034=CARTESIAN_POINT('Ctrl Pts',(79.5463978277233,-16.1917927772552,-1.62616608384562));
#32035=CARTESIAN_POINT('Ctrl Pts',(79.830336133723,-14.1196421847273,-8.84796354024379));
#32036=CARTESIAN_POINT('Ctrl Pts',(80.1785663678619,-7.2374943514207,-14.9946681804509));
#32037=CARTESIAN_POINT('Ctrl Pts',(80.5265809649815,1.84643761050977,-16.5367454191282));
#32038=CARTESIAN_POINT('Ctrl Pts',(80.8743817846602,10.3568459885564,-13.0118769647398));
#32039=CARTESIAN_POINT('Ctrl Pts',(81.2219788370638,15.6825995752614,-5.50309727131032));
#32040=CARTESIAN_POINT('Ctrl Pts',(81.5693820034866,16.197894141286,3.68117803479642));
#32041=CARTESIAN_POINT('Ctrl Pts',(81.9165951257598,11.7491068886896,11.7316901046367));
#32042=CARTESIAN_POINT('Ctrl Pts',(82.2250791599112,4.59879843509523,15.6763055088053));
#32043=CARTESIAN_POINT('Ctrl Pts',(82.494874661093,-2.38871229569965,15.9305201345378));
#32044=CARTESIAN_POINT('Ctrl Pts',(82.7260604745634,-8.04129839042069,13.9545033940471));
#32045=CARTESIAN_POINT('Ctrl Pts',(82.9571714599228,-12.5797889573595,10.0473605792937));
#32046=CARTESIAN_POINT('Ctrl Pts',(83.1882097228089,-15.3778215921963,4.75615357961634));
#32047=CARTESIAN_POINT('Ctrl Pts',(83.4191804497281,-16.0462077838481,-1.19082289641883));
#32048=CARTESIAN_POINT('Ctrl Pts',(83.6500940780417,-14.4978423341918,-6.96925130505314));
#32049=CARTESIAN_POINT('Ctrl Pts',(83.8809495762235,-10.9459258030931,-11.7814679381592));
#32050=CARTESIAN_POINT('Ctrl Pts',(84.1117286673162,-5.88383263291072,-14.963328438817));
#32051=CARTESIAN_POINT('Ctrl Pts',(84.3424712753825,-0.00960900109378653,
-16.0741042425561));
#32052=CARTESIAN_POINT('Ctrl Pts',(84.5731512945906,5.86267537367017,-14.9629860621253));
#32053=CARTESIAN_POINT('Ctrl Pts',(84.8037792961649,10.9218384506065,-11.7838260530281));
#32054=CARTESIAN_POINT('Ctrl Pts',(85.0343656809765,14.4698283252947,-6.97716202595678));
#32055=CARTESIAN_POINT('Ctrl Pts',(85.2648844583555,16.0144277219097,-1.2080918245963));
#32056=CARTESIAN_POINT('Ctrl Pts',(85.4953739959645,15.3458392252552,4.72610127787273));
#32057=CARTESIAN_POINT('Ctrl Pts',(85.7258198618693,12.5562210702063,10.00410823671));
#32058=CARTESIAN_POINT('Ctrl Pts',(85.9562252150393,8.0312146091608,13.8989981706252));
#32059=CARTESIAN_POINT('Ctrl Pts',(86.1865940423216,2.39864591071217,15.867693537978));
#32060=CARTESIAN_POINT('Ctrl Pts',(86.4553119485186,-4.56089462950754,15.6141613511442));
#32061=CARTESIAN_POINT('Ctrl Pts',(86.7623866182725,-11.6781310560641,11.6867952015708));
#32062=CARTESIAN_POINT('Ctrl Pts',(87.1077738505521,-16.1023612946132,3.67847646190086));
#32063=CARTESIAN_POINT('Ctrl Pts',(87.4531045042511,-15.5897167721347,-5.45112153800786));
#32064=CARTESIAN_POINT('Ctrl Pts',(87.7984014742918,-10.2975531213566,-12.908627927612));
#32065=CARTESIAN_POINT('Ctrl Pts',(88.1436343462562,-1.85181910129904,-16.4079507936403));
#32066=CARTESIAN_POINT('Ctrl Pts',(88.4889072862287,7.16466504256959,-14.8740297187205));
#32067=CARTESIAN_POINT('Ctrl Pts',(88.7764963641934,12.8387384302061,-9.80149223202101));
#32068=CARTESIAN_POINT('Ctrl Pts',(89.0067723369147,15.2512782914413,-4.38243329541124));
#32069=CARTESIAN_POINT('Ctrl Pts',(89.1216614258076,15.6621913514837,-1.49222289505446));
#32070=CARTESIAN_POINT('Ctrl Pts',(89.1793401389101,15.6649610610784,0.00157375857939028));
#32071=CARTESIAN_POINT('Ctrl Pts',(69.6184828603025,16.4616571598233,-0.030902239567753));
#32072=CARTESIAN_POINT('Ctrl Pts',(69.6789219655699,16.458754897209,1.53438465601481));
#32073=CARTESIAN_POINT('Ctrl Pts',(69.7997830801149,16.0266321943109,4.57501994136558));
#32074=CARTESIAN_POINT('Ctrl Pts',(70.0414349064678,13.4941722421641,10.2617903021912));
#32075=CARTESIAN_POINT('Ctrl Pts',(70.3432064666604,7.54051932200945,15.5847054098009));
#32076=CARTESIAN_POINT('Ctrl Pts',(70.7049768750637,-1.90873983484295,17.1894487135762));
#32077=CARTESIAN_POINT('Ctrl Pts',(71.0663492060979,-10.7475553396686,13.525924310196));
#32078=CARTESIAN_POINT('Ctrl Pts',(71.4273437518671,-16.2818464768058,5.72657424978343));
#32079=CARTESIAN_POINT('Ctrl Pts',(71.7278512234343,-16.7210289894503,-2.21659997283488));
#32080=CARTESIAN_POINT('Ctrl Pts',(71.9680675578449,-14.5106197428725,-7.98557322489482));
#32081=CARTESIAN_POINT('Ctrl Pts',(72.1481344157904,-11.7288725172833,-11.6852538002611));
#32082=CARTESIAN_POINT('Ctrl Pts',(72.328106524648,-8.03024824250695,-14.4669696417765));
#32083=CARTESIAN_POINT('Ctrl Pts',(72.5279702250768,-3.22977654241172,-16.300670274406));
#32084=CARTESIAN_POINT('Ctrl Pts',(72.7476856540044,2.4587525001183,-16.5141747132305));
#32085=CARTESIAN_POINT('Ctrl Pts',(72.9872078330289,8.31673840998305,-14.4634243432854));
#32086=CARTESIAN_POINT('Ctrl Pts',(73.2265632969346,13.0163496494046,-10.4182667032949));
#32087=CARTESIAN_POINT('Ctrl Pts',(73.4657526686465,15.9141590581627,-4.93897396144999));
#32088=CARTESIAN_POINT('Ctrl Pts',(73.7047766516472,16.6034312776959,1.21397241511146));
#32089=CARTESIAN_POINT('Ctrl Pts',(73.9834458021771,14.7409225736484,8.19195097348461));
#32090=CARTESIAN_POINT('Ctrl Pts',(74.301651818573,9.13086318160831,14.4766680019069));
#32091=CARTESIAN_POINT('Ctrl Pts',(74.6592672763964,0.0266353994119735,
17.0966775050227));
#32092=CARTESIAN_POINT('Ctrl Pts',(75.016519558125,-9.06348425632334,14.4765973593132));
#32093=CARTESIAN_POINT('Ctrl Pts',(75.3734117874807,-15.3610417662207,7.42742367726323));
#32094=CARTESIAN_POINT('Ctrl Pts',(75.7299471567895,-16.9418739975217,-1.88122771580553));
#32095=CARTESIAN_POINT('Ctrl Pts',(76.0861289312927,-13.3290621410899,-10.5975142741848));
#32096=CARTESIAN_POINT('Ctrl Pts',(76.4419606933661,-5.64617345782912,-16.0463992053949));
#32097=CARTESIAN_POINT('Ctrl Pts',(76.810612386967,4.11087115606672,-16.6005218369866));
#32098=CARTESIAN_POINT('Ctrl Pts',(77.0868204963524,10.4484384772329,-12.8295775485076));
#32099=CARTESIAN_POINT('Ctrl Pts',(77.3234199677928,14.1464940116618,-8.0565595801055));
#32100=CARTESIAN_POINT('Ctrl Pts',(77.5073642434964,16.0558684975652,-3.69288655028273));
#32101=CARTESIAN_POINT('Ctrl Pts',(77.743715642047,16.2835727900373,2.42892269363191));
#32102=CARTESIAN_POINT('Ctrl Pts',(77.9799198273595,14.2624210045081,8.20410639070391));
#32103=CARTESIAN_POINT('Ctrl Pts',(78.2159782861261,10.2721221270508,12.8404255794219));
#32104=CARTESIAN_POINT('Ctrl Pts',(78.451892297019,4.86870939460828,15.6955819848942));
#32105=CARTESIAN_POINT('Ctrl Pts',(78.687663274949,-1.20342672163651,16.3804065631851));
#32106=CARTESIAN_POINT('Ctrl Pts',(78.923292730736,-7.09646797598974,14.7976258939457));
#32107=CARTESIAN_POINT('Ctrl Pts',(79.1849474554113,-12.559397153018,10.7746599228106));
#32108=CARTESIAN_POINT('Ctrl Pts',(79.4202749429787,-15.5097121162534,5.34934186422077));
#32109=CARTESIAN_POINT('Ctrl Pts',(79.6946643695902,-16.3852200323318,-1.64037324259347));
#32110=CARTESIAN_POINT('Ctrl Pts',(79.9819403068823,-14.2884064522935,-8.94742064680176));
#32111=CARTESIAN_POINT('Ctrl Pts',(80.3342067288376,-7.3260467326971,-15.165426706738));
#32112=CARTESIAN_POINT('Ctrl Pts',(80.6861788812633,1.86167912032264,-16.7248261450382));
#32113=CARTESIAN_POINT('Ctrl Pts',(81.037862268153,10.4673895230379,-13.1602039003653));
#32114=CARTESIAN_POINT('Ctrl Pts',(81.3892625213115,15.8514527926196,-5.5687461546451));
#32115=CARTESIAN_POINT('Ctrl Pts',(81.7403859218982,16.3720606810702,3.71439472873355));
#32116=CARTESIAN_POINT('Ctrl Pts',(82.0912385240458,11.8761863054331,11.8495550298708));
#32117=CARTESIAN_POINT('Ctrl Pts',(82.4028723251709,4.65229996881944,15.8345467687591));
#32118=CARTESIAN_POINT('Ctrl Pts',(82.6753839687717,-2.4057965557233,16.0912478601411));
#32119=CARTESIAN_POINT('Ctrl Pts',(82.9088524431066,-8.11448174868296,14.0955831155642));
#32120=CARTESIAN_POINT('Ctrl Pts',(83.1422098352473,-12.6971950976412,10.1502287241044));
#32121=CARTESIAN_POINT('Ctrl Pts',(83.3754581634701,-15.522088392645,4.8081952387983));
#32122=CARTESIAN_POINT('Ctrl Pts',(83.6085992893649,-16.1966474690964,-1.19488542166675));
#32123=CARTESIAN_POINT('Ctrl Pts',(83.8416352233784,-14.6339538883274,-7.02670369688337));
#32124=CARTESIAN_POINT('Ctrl Pts',(84.0745679545012,-11.0497598473816,-11.8824317127295));
#32125=CARTESIAN_POINT('Ctrl Pts',(84.3073996737489,-5.94248428783527,-15.09263970399));
#32126=CARTESIAN_POINT('Ctrl Pts',(84.540132268385,-0.0171665032603614,
-16.2129461632812));
#32127=CARTESIAN_POINT('Ctrl Pts',(84.7727680106188,5.90520262635639,-15.0923025294507));
#32128=CARTESIAN_POINT('Ctrl Pts',(85.0053088744204,11.0065171159269,-11.8864785100097));
#32129=CARTESIAN_POINT('Ctrl Pts',(85.2377570340819,14.5833427924651,-7.04062680693156));
#32130=CARTESIAN_POINT('Ctrl Pts',(85.4701144791861,16.1401640578478,-1.22533588346504));
#32131=CARTESIAN_POINT('Ctrl Pts',(85.7023835299595,15.4662929248669,4.7550040735545));
#32132=CARTESIAN_POINT('Ctrl Pts',(85.9345662446591,12.6553888178413,10.0730373304554));
#32133=CARTESIAN_POINT('Ctrl Pts',(86.1666649327954,8.09679983295076,13.9966583914468));
#32134=CARTESIAN_POINT('Ctrl Pts',(86.3986815381799,2.42358552200963,15.9794357678464));
#32135=CARTESIAN_POINT('Ctrl Pts',(86.6692750541127,-4.58486198073758,15.7239726419428));
#32136=CARTESIAN_POINT('Ctrl Pts',(86.9783943834765,-11.7499252678846,11.7698005968098));
#32137=CARTESIAN_POINT('Ctrl Pts',(87.3259902517892,-16.2024151439095,3.70954956442589));
#32138=CARTESIAN_POINT('Ctrl Pts',(87.6734207471648,-15.6862303609498,-5.47622167055361));
#32139=CARTESIAN_POINT('Ctrl Pts',(88.0207132272952,-10.3628479251535,-12.9771513909202));
#32140=CARTESIAN_POINT('Ctrl Pts',(88.3678323138933,-1.8703041859877,-16.4954810466909));
#32141=CARTESIAN_POINT('Ctrl Pts',(88.7148821316246,7.193051660985,-14.9532751855446));
#32142=CARTESIAN_POINT('Ctrl Pts',(89.003856786706,12.8943942592402,-9.85553205895293));
#32143=CARTESIAN_POINT('Ctrl Pts',(89.2351907747089,15.3179503044652,-4.41141050395984));
#32144=CARTESIAN_POINT('Ctrl Pts',(89.3506074633962,15.7305922894428,-1.50774141983879));
#32145=CARTESIAN_POINT('Ctrl Pts',(89.4085387704217,15.7333741285005,-0.00740294277221285));
#32146=CARTESIAN_POINT('',(69.6184828603025,16.4616571598233,-0.0309022395677529));
#32147=CARTESIAN_POINT('Origin',(68.82,16.5,-1.31470342757595E-16));
#32148=CARTESIAN_POINT('',(89.4085387704217,15.7333741285004,-0.00740294277221266));
#32149=CARTESIAN_POINT('Ctrl Pts',(69.6184828603025,16.4616571598233,-0.030902239567753));
#32150=CARTESIAN_POINT('Ctrl Pts',(69.6789219655699,16.458754897209,1.53438465601481));
#32151=CARTESIAN_POINT('Ctrl Pts',(69.7997830801149,16.0266321943109,4.57501994136558));
#32152=CARTESIAN_POINT('Ctrl Pts',(70.0414349064678,13.4941722421641,10.2617903021912));
#32153=CARTESIAN_POINT('Ctrl Pts',(70.3432064666604,7.54051932200945,15.5847054098009));
#32154=CARTESIAN_POINT('Ctrl Pts',(70.7049768750637,-1.90873983484295,17.1894487135762));
#32155=CARTESIAN_POINT('Ctrl Pts',(71.0663492060979,-10.7475553396686,13.525924310196));
#32156=CARTESIAN_POINT('Ctrl Pts',(71.4273437518671,-16.2818464768058,5.72657424978343));
#32157=CARTESIAN_POINT('Ctrl Pts',(71.7278512234343,-16.7210289894503,-2.21659997283488));
#32158=CARTESIAN_POINT('Ctrl Pts',(71.9680675578449,-14.5106197428725,-7.98557322489482));
#32159=CARTESIAN_POINT('Ctrl Pts',(72.1481344157904,-11.7288725172833,-11.6852538002611));
#32160=CARTESIAN_POINT('Ctrl Pts',(72.328106524648,-8.03024824250695,-14.4669696417765));
#32161=CARTESIAN_POINT('Ctrl Pts',(72.5279702250768,-3.22977654241172,-16.300670274406));
#32162=CARTESIAN_POINT('Ctrl Pts',(72.7476856540044,2.4587525001183,-16.5141747132305));
#32163=CARTESIAN_POINT('Ctrl Pts',(72.9872078330289,8.31673840998305,-14.4634243432854));
#32164=CARTESIAN_POINT('Ctrl Pts',(73.2265632969346,13.0163496494046,-10.4182667032949));
#32165=CARTESIAN_POINT('Ctrl Pts',(73.4657526686465,15.9141590581627,-4.93897396144999));
#32166=CARTESIAN_POINT('Ctrl Pts',(73.7047766516472,16.6034312776959,1.21397241511146));
#32167=CARTESIAN_POINT('Ctrl Pts',(73.9834458021771,14.7409225736484,8.19195097348461));
#32168=CARTESIAN_POINT('Ctrl Pts',(74.301651818573,9.13086318160831,14.4766680019069));
#32169=CARTESIAN_POINT('Ctrl Pts',(74.6592672763964,0.0266353994119735,
17.0966775050227));
#32170=CARTESIAN_POINT('Ctrl Pts',(75.016519558125,-9.06348425632334,14.4765973593132));
#32171=CARTESIAN_POINT('Ctrl Pts',(75.3734117874807,-15.3610417662207,7.42742367726323));
#32172=CARTESIAN_POINT('Ctrl Pts',(75.7299471567895,-16.9418739975217,-1.88122771580553));
#32173=CARTESIAN_POINT('Ctrl Pts',(76.0861289312927,-13.3290621410899,-10.5975142741848));
#32174=CARTESIAN_POINT('Ctrl Pts',(76.4419606933661,-5.64617345782912,-16.0463992053949));
#32175=CARTESIAN_POINT('Ctrl Pts',(76.810612386967,4.11087115606672,-16.6005218369866));
#32176=CARTESIAN_POINT('Ctrl Pts',(77.0868204963524,10.4484384772329,-12.8295775485076));
#32177=CARTESIAN_POINT('Ctrl Pts',(77.3234199677928,14.1464940116618,-8.0565595801055));
#32178=CARTESIAN_POINT('Ctrl Pts',(77.5073642434964,16.0558684975652,-3.69288655028273));
#32179=CARTESIAN_POINT('Ctrl Pts',(77.743715642047,16.2835727900373,2.42892269363191));
#32180=CARTESIAN_POINT('Ctrl Pts',(77.9799198273595,14.2624210045081,8.20410639070391));
#32181=CARTESIAN_POINT('Ctrl Pts',(78.2159782861261,10.2721221270508,12.8404255794219));
#32182=CARTESIAN_POINT('Ctrl Pts',(78.451892297019,4.86870939460828,15.6955819848942));
#32183=CARTESIAN_POINT('Ctrl Pts',(78.687663274949,-1.20342672163651,16.3804065631851));
#32184=CARTESIAN_POINT('Ctrl Pts',(78.923292730736,-7.09646797598974,14.7976258939457));
#32185=CARTESIAN_POINT('Ctrl Pts',(79.1849474554113,-12.559397153018,10.7746599228106));
#32186=CARTESIAN_POINT('Ctrl Pts',(79.4202749429787,-15.5097121162534,5.34934186422077));
#32187=CARTESIAN_POINT('Ctrl Pts',(79.6946643695902,-16.3852200323318,-1.64037324259347));
#32188=CARTESIAN_POINT('Ctrl Pts',(79.9819403068823,-14.2884064522935,-8.94742064680176));
#32189=CARTESIAN_POINT('Ctrl Pts',(80.3342067288376,-7.3260467326971,-15.165426706738));
#32190=CARTESIAN_POINT('Ctrl Pts',(80.6861788812633,1.86167912032264,-16.7248261450382));
#32191=CARTESIAN_POINT('Ctrl Pts',(81.037862268153,10.4673895230379,-13.1602039003653));
#32192=CARTESIAN_POINT('Ctrl Pts',(81.3892625213115,15.8514527926196,-5.5687461546451));
#32193=CARTESIAN_POINT('Ctrl Pts',(81.7403859218982,16.3720606810702,3.71439472873355));
#32194=CARTESIAN_POINT('Ctrl Pts',(82.0912385240458,11.8761863054331,11.8495550298708));
#32195=CARTESIAN_POINT('Ctrl Pts',(82.4028723251709,4.65229996881944,15.8345467687591));
#32196=CARTESIAN_POINT('Ctrl Pts',(82.6753839687717,-2.4057965557233,16.0912478601411));
#32197=CARTESIAN_POINT('Ctrl Pts',(82.9088524431066,-8.11448174868296,14.0955831155642));
#32198=CARTESIAN_POINT('Ctrl Pts',(83.1422098352473,-12.6971950976412,10.1502287241044));
#32199=CARTESIAN_POINT('Ctrl Pts',(83.3754581634701,-15.522088392645,4.8081952387983));
#32200=CARTESIAN_POINT('Ctrl Pts',(83.6085992893649,-16.1966474690964,-1.19488542166675));
#32201=CARTESIAN_POINT('Ctrl Pts',(83.8416352233784,-14.6339538883274,-7.02670369688337));
#32202=CARTESIAN_POINT('Ctrl Pts',(84.0745679545012,-11.0497598473816,-11.8824317127295));
#32203=CARTESIAN_POINT('Ctrl Pts',(84.3073996737489,-5.94248428783527,-15.09263970399));
#32204=CARTESIAN_POINT('Ctrl Pts',(84.540132268385,-0.0171665032603614,
-16.2129461632812));
#32205=CARTESIAN_POINT('Ctrl Pts',(84.7727680106188,5.90520262635639,-15.0923025294507));
#32206=CARTESIAN_POINT('Ctrl Pts',(85.0053088744204,11.0065171159269,-11.8864785100097));
#32207=CARTESIAN_POINT('Ctrl Pts',(85.2377570340819,14.5833427924651,-7.04062680693156));
#32208=CARTESIAN_POINT('Ctrl Pts',(85.4701144791861,16.1401640578478,-1.22533588346504));
#32209=CARTESIAN_POINT('Ctrl Pts',(85.7023835299595,15.4662929248669,4.7550040735545));
#32210=CARTESIAN_POINT('Ctrl Pts',(85.9345662446591,12.6553888178413,10.0730373304554));
#32211=CARTESIAN_POINT('Ctrl Pts',(86.1666649327954,8.09679983295076,13.9966583914468));
#32212=CARTESIAN_POINT('Ctrl Pts',(86.3986815381799,2.42358552200963,15.9794357678464));
#32213=CARTESIAN_POINT('Ctrl Pts',(86.6692750541127,-4.58486198073758,15.7239726419428));
#32214=CARTESIAN_POINT('Ctrl Pts',(86.9783943834765,-11.7499252678846,11.7698005968098));
#32215=CARTESIAN_POINT('Ctrl Pts',(87.3259902517892,-16.2024151439095,3.70954956442589));
#32216=CARTESIAN_POINT('Ctrl Pts',(87.6734207471648,-15.6862303609498,-5.47622167055361));
#32217=CARTESIAN_POINT('Ctrl Pts',(88.0207132272952,-10.3628479251535,-12.9771513909202));
#32218=CARTESIAN_POINT('Ctrl Pts',(88.3678323138933,-1.8703041859877,-16.4954810466909));
#32219=CARTESIAN_POINT('Ctrl Pts',(88.7148821316246,7.193051660985,-14.9532751855446));
#32220=CARTESIAN_POINT('Ctrl Pts',(89.003856786706,12.8943942592402,-9.85553205895293));
#32221=CARTESIAN_POINT('Ctrl Pts',(89.2351907747089,15.3179503044652,-4.41141050395984));
#32222=CARTESIAN_POINT('Ctrl Pts',(89.3506074633962,15.7305922894428,-1.50774141983879));
#32223=CARTESIAN_POINT('Ctrl Pts',(89.4085387704217,15.7333741285005,-0.00740294277221285));
#32224=CARTESIAN_POINT('Origin',(89.18,16.5,-1.97064586870965E-14));
#32225=CARTESIAN_POINT('Origin',(89.18,16.5,-1.97064586870965E-14));
#32226=CARTESIAN_POINT('Origin',(68.82,16.5,-1.31470342757595E-16));
#45197=UNCERTAINTY_MEASURE_WITH_UNIT(LENGTH_MEASURE(0.01),#45237,
'DISTANCE_ACCURACY_VALUE',
'Maximum model space distance between geometric entities at asserted c
onnectivities');
#45214=UNCERTAINTY_MEASURE_WITH_UNIT(LENGTH_MEASURE(0.01),#45237,
'DISTANCE_ACCURACY_VALUE',
'Maximum model space distance between geometric entities at asserted c
onnectivities');
#45219=(
GEOMETRIC_REPRESENTATION_CONTEXT(3)
GLOBAL_UNCERTAINTY_ASSIGNED_CONTEXT((#45197))
GLOBAL_UNIT_ASSIGNED_CONTEXT((#45237,#45239,#45240))
REPRESENTATION_CONTEXT('','3D')
);
#45236=(
GEOMETRIC_REPRESENTATION_CONTEXT(3)
GLOBAL_UNCERTAINTY_ASSIGNED_CONTEXT((#45214))
GLOBAL_UNIT_ASSIGNED_CONTEXT((#45237,#45239,#45240))
REPRESENTATION_CONTEXT('','3D')
);
#45237=(
LENGTH_UNIT()
NAMED_UNIT(*)
SI_UNIT(.MILLI.,.METRE.)
);
#45239=(
NAMED_UNIT(*)
PLANE_ANGLE_UNIT()
SI_UNIT($,.RADIAN.)
);
#45240=(
NAMED_UNIT(*)
SI_UNIT($,.STERADIAN.)
SOLID_ANGLE_UNIT()
);
#45245=SHAPE_DEFINITION_REPRESENTATION(#45266,#45317);
#45266=PRODUCT_DEFINITION_SHAPE('',$,#45339);
#45317=SHAPE_REPRESENTATION('',(#17147),#45219);
#45334=PRODUCT_DEFINITION_CONTEXT('part definition',#45399,'design');
#45339=PRODUCT_DEFINITION('2026-10-25-23-38-15-879',
'04_Piston_Return_Spring_D33x1.6',#45360,#45334);
#45360=PRODUCT_DEFINITION_FORMATION('',$,#45405);
#45399=APPLICATION_CONTEXT(
'Core Data for Automotive Mechanical Design Process');
#45400=PRODUCT_CONTEXT('part definition',#45399,'mechanical');
#45405=PRODUCT('2026-10-25-23-38-15-879',
'04_Piston_Return_Spring_D33x1.6',$,(#45400));
#45478=COLOUR_RGB('Grey',0.48,0.52,0.57);
#45479=FILL_AREA_STYLE_COLOUR('',#45478);
#45480=FILL_AREA_STYLE('',(#45479));
#45481=SURFACE_STYLE_FILL_AREA(#45480);
#45482=SURFACE_SIDE_STYLE('',(#45481));
#45483=SURFACE_STYLE_USAGE(.BOTH.,#45482);
#45484=PRESENTATION_STYLE_ASSIGNMENT((#45483));
ENDSEC;
END-ISO-10303-21;
